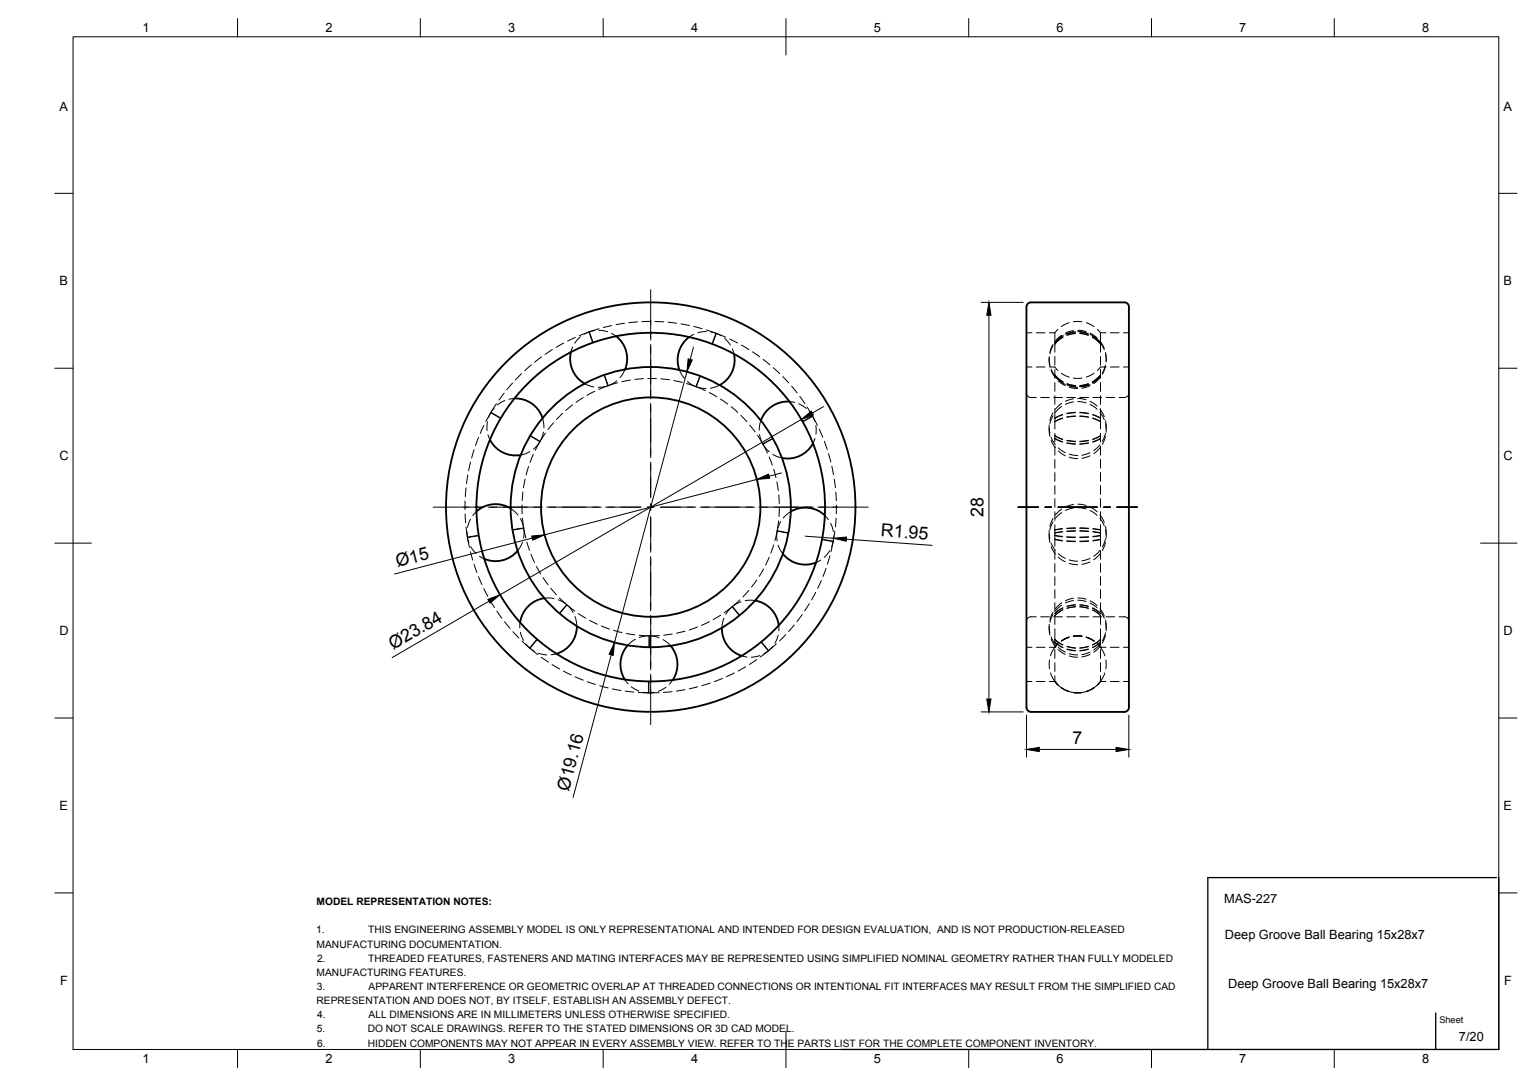
ISO-10303-21;
HEADER;
FILE_DESCRIPTION (('STEP AP214'),
    '1' );
FILE_NAME ( 'Deep Groove Ball Bearing 15x28x7.step', '2026-10-06T08:24:41', ( '' ), ( '' ), 'STEP AP214', 'Unspecified', '' );
FILE_SCHEMA (( 'AUTOMOTIVE_DESIGN' ));
ENDSEC;
DATA;
#5=EDGE_CURVE ( 'NONE', #3462, #12596, #11883, .T. ) ;
#6=CARTESIAN_POINT ( 'NONE',  ( 0.3607825703614780388, 0.06309631803704385256, 0.08455817587619855746 ) ) ;
#11=ORIENTED_EDGE ( 'NONE', *, *, #14941, .F. ) ;
#36=CARTESIAN_POINT ( 'NONE',  ( 0.4620608682196346573, 0.08206165078060492779, 0.1992125984251968684 ) ) ;
#61=AXIS2_PLACEMENT_3D ( 'NONE', #22056, #14008, #15706 ) ;
#62=CARTESIAN_POINT ( 'NONE',  ( 0.2428345617565153547, 0.2885915454824177218, 0.1992125984251968684 ) ) ;
#79=EDGE_LOOP ( 'NONE', ( #24549, #12991, #16155, #19629, #1630 ) ) ;
#92=DIRECTION ( 'NONE',  ( -0.8660254037844387076, 0.4999999999999998890, 0.000000000000000000 ) ) ;
#96=ORIENTED_EDGE ( 'NONE', *, *, #21914, .F. ) ;
#100=PRODUCT_DEFINITION_CONTEXT ( 'detailed design', #9805, 'design' ) ;
#103=CARTESIAN_POINT ( 'NONE',  ( 0.1669771619554775988, -0.4570419016558947556, 0.1827409795206137999 ) ) ;
#108=EDGE_LOOP ( 'NONE', ( #16831, #22102, #23011, #14973, #23434 ) ) ;
#112=AXIS2_PLACEMENT_3D ( 'NONE', #26701, #7362, #3107 ) ;
#125=DIRECTION ( 'NONE',  ( 0.000000000000000000, -1.000000000000000000, 0.000000000000000000 ) ) ;
#126=CARTESIAN_POINT ( 'NONE',  ( 0.0005789221761808661720, 0.4692909815006409691, 0.1992125984251968684 ) ) ;
#128=CARTESIAN_POINT ( 'NONE',  ( 0.000000000000000000, 0.000000000000000000, 0.01181102362204724393 ) ) ;
#135=ORIENTED_EDGE ( 'NONE', *, *, #15589, .F. ) ;
#137=DIRECTION ( 'NONE',  ( 0.000000000000000000, 0.000000000000000000, 1.000000000000000000 ) ) ;
#165=CARTESIAN_POINT ( 'NONE',  ( 0.000000000000000000, 0.000000000000000000, -3.278217716535432842E-17 ) ) ;
#169=EDGE_CURVE ( 'NONE', #21708, #16172, #21378, .T. ) ;
#182=CIRCLE ( 'NONE', #19069, 0.2952755905511810774 ) ;
#186=B_SPLINE_CURVE_WITH_KNOTS ( 'NONE', 3,
 ( #3405, #6229, #8475, #4376, #23337, #25576 ),
 .UNSPECIFIED., .F., .F.,
 ( 4, 2, 4 ),
 ( 0.2291966065698869959, 0.2305109203526899964, 0.2318252341354939960 ),
 .UNSPECIFIED. ) ;
#199=CARTESIAN_POINT ( 'NONE',  ( -0.3665264996331779601, -0.2116141732283464416, 0.1377952755905511861 ) ) ;
#211=EDGE_CURVE ( 'NONE', #8069, #8578, #17150, .T. ) ;
#222=SURFACE_STYLE_USAGE ( .BOTH. , #19537 ) ;
#226=CARTESIAN_POINT ( 'NONE',  ( 0.0005189969344232283309, 0.3771649972486724733, 0.07637795275590551769 ) ) ;
#230=ADVANCED_FACE ( 'NONE', ( #18229 ), #8731, .T. ) ;
#235=EDGE_CURVE ( 'NONE', #27620, #935, #8316, .T. ) ;
#237=FACE_OUTER_BOUND ( 'NONE', #646, .T. ) ;
#240=VERTEX_POINT ( 'NONE', #18659 ) ;
#243=FACE_OUTER_BOUND ( 'NONE', #27157, .T. ) ;
#251=EDGE_CURVE ( 'NONE', #10904, #1560, #4337, .T. ) ;
#256=DIRECTION ( 'NONE',  ( 0.000000000000000000, 0.000000000000000000, 1.000000000000000000 ) ) ;
#263=ORIENTED_EDGE ( 'NONE', *, *, #3631, .F. ) ;
#266=CIRCLE ( 'NONE', #11488, 0.4692913385826771866 ) ;
#286=B_SPLINE_CURVE_WITH_KNOTS ( 'NONE', 3,
 ( #23808, #10659, #8682, #25644, #1905, #25921 ),
 .UNSPECIFIED., .F., .F.,
 ( 4, 2, 4 ),
 ( 0.7157687286427140139, 0.7172350147555670574, 0.7187013008684199900 ),
 .UNSPECIFIED. ) ;
#308=DIRECTION ( 'NONE',  ( 0.7660444431189782355, 0.6427876096865391409, 0.000000000000000000 ) ) ;
#309=( CONVERSION_BASED_UNIT ( 'INCH', #689 ) LENGTH_UNIT ( ) NAMED_UNIT ( #9238 ) ) ;
#326=CARTESIAN_POINT ( 'NONE',  ( -0.1196556571310431333, -0.3272932875252256291, 0.1166443193928402983 ) ) ;
#339=VERTEX_POINT ( 'NONE', #12317 ) ;
#343=DIRECTION ( 'NONE',  ( 0.000000000000000000, 1.000000000000000000, 0.000000000000000000 ) ) ;
#355=EDGE_CURVE ( 'NONE', #14294, #8859, #26577, .T. ) ;
#365=CARTESIAN_POINT ( 'NONE',  ( 0.3411065095061437402, 0.06065137456822566192, 0.1377952755905510474 ) ) ;
#366=DIRECTION ( 'NONE',  ( 0.000000000000000000, 1.000000000000000000, 0.000000000000000000 ) ) ;
#367=AXIS2_PLACEMENT_3D ( 'NONE', #8300, #14535, #6190 ) ;
#370=ORIENTED_EDGE ( 'NONE', *, *, #13419, .F. ) ;
#385=CARTESIAN_POINT ( 'NONE',  ( -0.2230788859036006988, 0.2650812153444457309, 0.1276989850646860214 ) ) ;
#387=ORIENTED_EDGE ( 'NONE', *, *, #3265, .F. ) ;
#391=AXIS2_PLACEMENT_3D ( 'NONE', #18400, #12341, #14636 ) ;
#394=LINE ( 'NONE', #15375, #16281 ) ;
#404=VECTOR ( 'NONE', #11672, 39.37007874015748143 ) ;
#420=CARTESIAN_POINT ( 'NONE',  ( 0.3002886982018041495, -0.1727973894384573217, 0.1478915661278440430 ) ) ;
#421=TOROIDAL_SURFACE ( 'NONE', #8530, 0.4232283464566928832, 0.07677165354330708902 ) ;
#429=CIRCLE ( 'NONE', #27509, 0.07677362204724409722 ) ;
#435=DIRECTION ( 'NONE',  ( 0.000000000000000000, -1.000000000000000000, 0.000000000000000000 ) ) ;
#449=CARTESIAN_POINT ( 'NONE',  ( 0.3665264996331779601, -0.2116141732283464416, 0.06102165354330708891 ) ) ;
#451=CARTESIAN_POINT ( 'NONE',  ( 0.0003854097503897235258, 0.4692912202195575477, 0.07637630773773071424 ) ) ;
#457=AXIS2_PLACEMENT_3D ( 'NONE', #11632, #18253, #20541 ) ;
#484=CARTESIAN_POINT ( 'NONE',  ( 0.1706130639257694703, -0.4670119966460608563, 0.1140743250952255261 ) ) ;
#496=VERTEX_POINT ( 'NONE', #19091 ) ;
#497=CIRCLE ( 'NONE', #20352, 0.4692913385826771866 ) ;
#500=B_SPLINE_CURVE_WITH_KNOTS ( 'NONE', 3,
 ( #10699, #21447, #8173, #14554, #4212, #19314, #8315, #6201, #17200, #2088 ),
 .UNSPECIFIED., .F., .F.,
 ( 4, 2, 2, 2, 4 ),
 ( 0.000000000000000000, 0.2500000000000000000, 0.5000000000000000000, 0.7500000000000000000, 1.000000000000000000 ),
 .UNSPECIFIED. ) ;
#509=ADVANCED_FACE ( 'NONE', ( #25741, #6394 ), #27730, .T. ) ;
#515=DIRECTION ( 'NONE',  ( 0.000000000000000000, 1.000000000000000000, 0.000000000000000000 ) ) ;
#516=SHAPE_DEFINITION_REPRESENTATION ( #3947, #26684 ) ;
#551=CARTESIAN_POINT ( 'NONE',  ( 0.4061284506584276199, -0.2351468520616558922, 0.07637795275590551769 ) ) ;
#552=ORIENTED_EDGE ( 'NONE', *, *, #3585, .T. ) ;
#555=CARTESIAN_POINT ( 'NONE',  ( -0.4792984784078200833, 0.08391448672304414880, 0.09284957166327162392 ) ) ;
#559=CARTESIAN_POINT ( 'NONE',  ( -0.2420394123212937232, 0.2892587550802429575, 0.1992125984251968684 ) ) ;
#567=DIRECTION ( 'NONE',  ( 0.000000000000000000, 1.000000000000000000, 0.000000000000000000 ) ) ;
#573=FACE_BOUND ( 'NONE', #23313, .T. ) ;
#575=B_SPLINE_CURVE_WITH_KNOTS ( 'NONE', 3,
 ( #21559, #25522, #19016, #21142, #6187, #25800, #4193, #19296, #10823, #27882 ),
 .UNSPECIFIED., .F., .F.,
 ( 4, 2, 2, 2, 4 ),
 ( 0.000000000000000000, 0.2500000000000000000, 0.5000000000000000000, 0.7500000000000000000, 1.000000000000000000 ),
 .UNSPECIFIED. ) ;
#582=CARTESIAN_POINT ( 'NONE',  ( -0.1291602287245499914, -0.3543605079199910191, 0.07637549214372835182 ) ) ;
#584=DIRECTION ( 'NONE',  ( 0.000000000000000000, 0.000000000000000000, 1.000000000000000000 ) ) ;
#586=CIRCLE ( 'NONE', #13192, 0.3464566929133857665 ) ;
#596=B_SPLINE_CURVE_WITH_KNOTS ( 'NONE', 3,
 ( #25551, #6069, #1950, #3792, #12413, #10279 ),
 .UNSPECIFIED., .F., .F.,
 ( 4, 2, 4 ),
 ( 0.6902184472752670441, 0.6915327610580710438, 0.6928470748408740443 ),
 .UNSPECIFIED. ) ;
#602=CARTESIAN_POINT ( 'NONE',  ( 0.000000000000000000, 0.000000000000000000, 0.2637795275590551491 ) ) ;
#604=CARTESIAN_POINT ( 'NONE',  ( -0.4302903874076512425, -0.2491168502841591137, 0.1615162260931827798 ) ) ;
#608=EDGE_CURVE ( 'NONE', #21708, #2190, #18099, .T. ) ;
#610=CARTESIAN_POINT ( 'NONE',  ( 0.0005114926878545973925, 0.3662580330867914458, 0.1910323753037862504 ) ) ;
#613=CARTESIAN_POINT ( 'NONE',  ( 0.3714952424334504455, 0.06515381386493819538, 0.1992142436757342316 ) ) ;
#634=CARTESIAN_POINT ( 'NONE',  ( 0.3665264996331779601, -0.2116141732283464416, 0.2145688976377952695 ) ) ;
#635=ADVANCED_FACE ( 'NONE', ( #22183 ), #9450, .T. ) ;
#646=EDGE_LOOP ( 'NONE', ( #20143, #20285, #18872, #16802, #20608, #22874 ) ) ;
#658=ORIENTED_EDGE ( 'NONE', *, *, #21103, .T. ) ;
#661=VERTEX_POINT ( 'NONE', #24573 ) ;
#676=EDGE_CURVE ( 'NONE', #25669, #5138, #6693, .T. ) ;
#678=DIRECTION ( 'NONE',  ( 0.000000000000000000, 0.000000000000000000, 1.000000000000000000 ) ) ;
#687=AXIS2_PLACEMENT_3D ( 'NONE', #19653, #20189, #4936 ) ;
#689=LENGTH_MEASURE_WITH_UNIT ( LENGTH_MEASURE( 0.02539999999999999897 ), #14996 ) ;
#690=ORIENTED_EDGE ( 'NONE', *, *, #10619, .F. ) ;
#710=AXIS2_PLACEMENT_3D ( 'NONE', #24848, #16245, #9579 ) ;
#729=DIRECTION ( 'NONE',  ( 0.000000000000000000, 1.000000000000000000, 0.000000000000000000 ) ) ;
#735=CARTESIAN_POINT ( 'NONE',  ( 0.1447526197146039584, -0.3977045540727763839, 0.2145688976377952695 ) ) ;
#740=ORIENTED_EDGE ( 'NONE', *, *, #20229, .T. ) ;
#762=VERTEX_POINT ( 'NONE', #16114 ) ;
#764=VERTEX_POINT ( 'NONE', #8065 ) ;
#788=AXIS2_PLACEMENT_3D ( 'NONE', #5285, #22529, #17715 ) ;
#803=ORIENTED_EDGE ( 'NONE', *, *, #20955, .T. ) ;
#812=DIRECTION ( 'NONE',  ( 1.000000000000000000, 0.000000000000000000, 0.000000000000000000 ) ) ;
#820=DIRECTION ( 'NONE',  ( -0.9848077530122079093, 0.1736481776669309696, 0.000000000000000000 ) ) ;
#834=CARTESIAN_POINT ( 'NONE',  ( -0.4065144339881236468, -0.2344790234878192936, 0.07637549214372835182 ) ) ;
#835=ORIENTED_EDGE ( 'NONE', *, *, #3265, .T. ) ;
#845=CARTESIAN_POINT ( 'NONE',  ( 0.000000000000000000, 0.3771653543307086909, 0.2755905511811023723 ) ) ;
#848=DIRECTION ( 'NONE',  ( 0.000000000000000000, 0.000000000000000000, 1.000000000000000000 ) ) ;
#854=CARTESIAN_POINT ( 'NONE',  ( -0.1180276236025431108, -0.3257325899126714552, 0.1276989850612303967 ) ) ;
#881=ORIENTED_EDGE ( 'NONE', *, *, #14494, .F. ) ;
#884=CARTESIAN_POINT ( 'NONE',  ( -0.3105951325225213000, -0.1787383246545907467, 0.09506557084360875431 ) ) ;
#890=CARTESIAN_POINT ( 'NONE',  ( -0.3714653163189441387, 0.06532421472592696288, 0.07637549214372835182 ) ) ;
#916=DIRECTION ( 'NONE',  ( 0.000000000000000000, 0.000000000000000000, -1.000000000000000000 ) ) ;
#935=VERTEX_POINT ( 'NONE', #19202 ) ;
#946=EDGE_LOOP ( 'NONE', ( #5245, #370, #4472, #8238, #9152, #16696 ) ) ;
#954=DIRECTION ( 'NONE',  ( 0.000000000000000000, 1.000000000000000000, 0.000000000000000000 ) ) ;
#959=CARTESIAN_POINT ( 'NONE',  ( -0.4062254136079196942, -0.2349793847445165174, 0.1992142434433712694 ) ) ;
#986=CARTESIAN_POINT ( 'NONE',  ( 0.2230788859036007821, 0.2650812153444456198, 0.1377952755905513527 ) ) ;
#994=CARTESIAN_POINT ( 'NONE',  ( -0.1187185187216169419, -0.3276343780110584913, 0.1166443193947863527 ) ) ;
#997=DIRECTION ( 'NONE',  ( 0.000000000000000000, 0.000000000000000000, 1.000000000000000000 ) ) ;
#998=CARTESIAN_POINT ( 'NONE',  ( -0.3012109481301850633, 0.3598698725862389813, 0.07637795275590551769 ) ) ;
#1006=AXIS2_PLACEMENT_3D ( 'NONE', #24971, #1119, #11840 ) ;
#1036=CARTESIAN_POINT ( 'NONE',  ( 0.000000000000000000, 0.000000000000000000, 0.1992125984251968684 ) ) ;
#1049=CARTESIAN_POINT ( 'NONE',  ( -0.0003454908279975151160, 0.3771652360013086902, 0.07637630750536809898 ) ) ;
#1050=ORIENTED_EDGE ( 'NONE', *, *, #16246, .F. ) ;
#1055=FACE_BOUND ( 'NONE', #16566, .T. ) ;
#1085=VERTEX_POINT ( 'NONE', #2918 ) ;
#1119=DIRECTION ( 'NONE',  ( 0.3420201433256691570, 0.9396926207859084279, -0.000000000000000000 ) ) ;
#1122=EDGE_LOOP ( 'NONE', ( #10970, #9534, #26213, #4529, #19127, #25779 ) ) ;
#1134=EDGE_CURVE ( 'NONE', #2754, #5280, #13734, .T. ) ;
#1137=B_SPLINE_CURVE_WITH_KNOTS ( 'NONE', 3,
 ( #26836, #22317, #13559, #16110, #2949, #11581, #1140, #9447, #18338, #998 ),
 .UNSPECIFIED., .F., .F.,
 ( 4, 2, 2, 2, 4 ),
 ( 0.000000000000000000, 0.2500000000000000000, 0.5000000000000000000, 0.7500000000000000000, 1.000000000000000000 ),
 .UNSPECIFIED. ) ;
#1140=CARTESIAN_POINT ( 'NONE',  ( -0.3191377210036941414, 0.3812612458990542463, 0.1140743250907937795 ) ) ;
#1166=CARTESIAN_POINT ( 'NONE',  ( 0.000000000000000000, 0.000000000000000000, 0.1377952755905511584 ) ) ;
#1171=CARTESIAN_POINT ( 'NONE',  ( -0.1285103288269285327, -0.3545966721392122545, 0.1992125984251968684 ) ) ;
#1174=CARTESIAN_POINT ( 'NONE',  ( 0.1601448837025507554, -0.4411213145380000200, 0.07637630773773071424 ) ) ;
#1179=TOROIDAL_SURFACE ( 'NONE', #8830, 0.4232283464566928832, 0.07677165354330708902 ) ;
#1199=DIRECTION ( 'NONE',  ( -0.6427876096865393629, 0.7660444431189780135, 0.000000000000000000 ) ) ;
#1201=CARTESIAN_POINT ( 'NONE',  ( -0.2420394123212937232, 0.2892587550802429575, 0.1992125984251968684 ) ) ;
#1213=CARTESIAN_POINT ( 'NONE',  ( 0.000000000000000000, 0.000000000000000000, 0.2374015748031496065 ) ) ;
#1218=AXIS2_PLACEMENT_3D ( 'NONE', #22516, #18393, #22374 ) ;
#1219=EDGE_CURVE ( 'NONE', #15450, #13929, #14689, .T. ) ;
#1238=CARTESIAN_POINT ( 'NONE',  ( 0.2952755905511810774, 0.000000000000000000, 0.2637795275590551491 ) ) ;
#1247=LINE ( 'NONE', #7602, #6111 ) ;
#1255=CARTESIAN_POINT ( 'NONE',  ( 0.000000000000000000, 0.000000000000000000, 0.01181102362204724393 ) ) ;
#1273=CARTESIAN_POINT ( 'NONE',  ( 0.4167985568850881561, 0.07349283109919289847, 0.06102165354330708891 ) ) ;
#1284=ORIENTED_EDGE ( 'NONE', *, *, #15743, .T. ) ;
#1290=FACE_OUTER_BOUND ( 'NONE', #17007, .T. ) ;
#1306=CARTESIAN_POINT ( 'NONE',  ( 0.2421724791772047192, 0.2891474103999575052, 0.1992142436757342316 ) ) ;
#1318=ADVANCED_FACE ( 'NONE', ( #14391 ), #2030, .T. ) ;
#1324=CARTESIAN_POINT ( 'NONE',  ( -0.3002886982018051487, -0.1727973894384558229, 0.1377952755905512416 ) ) ;
#1327=ORIENTED_EDGE ( 'NONE', *, *, #24883, .T. ) ;
#1333=CARTESIAN_POINT ( 'NONE',  ( -0.2350342994822195442, 0.2808987121525407527, 0.1910323753003855540 ) ) ;
#1348=VERTEX_POINT ( 'NONE', #21008 ) ;
#1350=FACE_OUTER_BOUND ( 'NONE', #24867, .T. ) ;
#1352=ORIENTED_EDGE ( 'NONE', *, *, #11882, .T. ) ;
#1361=B_SPLINE_CURVE_WITH_KNOTS ( 'NONE', 3,
 ( #7535, #1049, #3140, #9640 ),
 .UNSPECIFIED., .F., .F.,
 ( 4, 4 ),
 ( 0.2291966065698869959, 0.2305109203526903294 ),
 .UNSPECIFIED. ) ;
#1371=EDGE_CURVE ( 'NONE', #12126, #25040, #6106, .T. ) ;
#1392=CARTESIAN_POINT ( 'NONE',  ( -0.3715251363271980245, 0.06498290224717540031, 0.1992125984251968684 ) ) ;
#1394=CARTESIAN_POINT ( 'NONE',  ( 0.4620608682196346573, 0.08206165078060492779, 0.1992125984251968684 ) ) ;
#1409=EDGE_CURVE ( 'NONE', #18722, #9569, #7421, .T. ) ;
#1414=DIRECTION ( 'NONE',  ( 1.000000000000000000, 0.000000000000000000, 0.000000000000000000 ) ) ;
#1415=EDGE_CURVE ( 'NONE', #3132, #19812, #19791, .T. ) ;
#1420=CARTESIAN_POINT ( 'NONE',  ( 0.000000000000000000, 0.000000000000000000, 0.1377952755905511861 ) ) ;
#1424=CARTESIAN_POINT ( 'NONE',  ( -0.0005963271530280589861, 0.4972008316414383566, 0.1615162260929405846 ) ) ;
#1431=EDGE_CURVE ( 'NONE', #19638, #3330, #1584, .T. ) ;
#1457=CARTESIAN_POINT ( 'NONE',  ( 0.2350342994834856425, 0.2808987121540589826, 0.08455817587923418477 ) ) ;
#1477=ORIENTED_EDGE ( 'NONE', *, *, #1134, .F. ) ;
#1480=CARTESIAN_POINT ( 'NONE',  ( 0.3715251363271980245, 0.06498290224717499786, 0.1992125984251968684 ) ) ;
#1500=DIRECTION ( 'NONE',  ( 0.000000000000000000, 0.000000000000000000, 1.000000000000000000 ) ) ;
#1511=ORIENTED_EDGE ( 'NONE', *, *, #15544, .T. ) ;
#1517=DIRECTION ( 'NONE',  ( 0.000000000000000000, 0.000000000000000000, -1.000000000000000000 ) ) ;
#1518=DIRECTION ( 'NONE',  ( 0.000000000000000000, 0.000000000000000000, 1.000000000000000000 ) ) ;
#1519=DIRECTION ( 'NONE',  ( 0.000000000000000000, 0.000000000000000000, 1.000000000000000000 ) ) ;
#1524=ORIENTED_EDGE ( 'NONE', *, *, #26785, .T. ) ;
#1535=EDGE_CURVE ( 'NONE', #4856, #13865, #15573, .T. ) ;
#1540=CARTESIAN_POINT ( 'NONE',  ( 0.0004974201395668343718, 0.3464563358313495489, 0.1276989850566408180 ) ) ;
#1554=EDGE_LOOP ( 'NONE', ( #11117, #19270 ) ) ;
#1559=DIRECTION ( 'NONE',  ( 1.224646799147353207E-16, 1.000000000000000000, -0.000000000000000000 ) ) ;
#1560=VERTEX_POINT ( 'NONE', #19724 ) ;
#1566=DIRECTION ( 'NONE',  ( 0.000000000000000000, 0.000000000000000000, -1.000000000000000000 ) ) ;
#1573=ORIENTED_EDGE ( 'NONE', *, *, #16459, .T. ) ;
#1584=CIRCLE ( 'NONE', #6558, 0.4692913385826771866 ) ;
#1588=AXIS2_PLACEMENT_3D ( 'NONE', #21238, #19108, #17001 ) ;
#1593=DIRECTION ( 'NONE',  ( 0.000000000000000000, 1.000000000000000000, 0.000000000000000000 ) ) ;
#1614=CIRCLE ( 'NONE', #25063, 0.3771653543307086909 ) ;
#1630=ORIENTED_EDGE ( 'NONE', *, *, #18890, .F. ) ;
#1637=VERTEX_POINT ( 'NONE', #16323 ) ;
#1640=DIRECTION ( 'NONE',  ( -0.1736481776669300814, 0.9848077530122080203, 0.000000000000000000 ) ) ;
#1648=CARTESIAN_POINT ( 'NONE',  ( 0.3191377210044040735, 0.3812612458998947962, 0.1140743250939253023 ) ) ;
#1660=EDGE_LOOP ( 'NONE', ( #6013, #15520, #22967, #15519, #15320, #14141, #22628, #12183, #8642, #1327, #3586, #8439, #26231 ) ) ;
#1661=AXIS2_PLACEMENT_3D ( 'NONE', #6156, #15392, #11060 ) ;
#1663=DIRECTION ( 'NONE',  ( 1.000000000000000000, 0.000000000000000000, 0.000000000000000000 ) ) ;
#1683=CARTESIAN_POINT ( 'NONE',  ( 0.000000000000000000, 0.4232283464566928832, 0.2755905511811023723 ) ) ;
#1705=DIRECTION ( 'NONE',  ( 0.000000000000000000, 0.000000000000000000, 1.000000000000000000 ) ) ;
#1737=ORIENTED_EDGE ( 'NONE', *, *, #24013, .T. ) ;
#1787=DIRECTION ( 'NONE',  ( 0.000000000000000000, 1.000000000000000000, 0.000000000000000000 ) ) ;
#1793=FACE_OUTER_BOUND ( 'NONE', #6745, .T. ) ;
#1798=CARTESIAN_POINT ( 'NONE',  ( -0.3019498226894488102, 0.3592501948414881796, 0.07637630773773090853 ) ) ;
#1799=DIRECTION ( 'NONE',  ( 0.000000000000000000, 0.000000000000000000, 1.000000000000000000 ) ) ;
#1801=EDGE_LOOP ( 'NONE', ( #9800, #18373 ) ) ;
#1811=ORIENTED_EDGE ( 'NONE', *, *, #169, .T. ) ;
#1819=CARTESIAN_POINT ( 'NONE',  ( 0.000000000000000000, 0.000000000000000000, 0.1992125984251968684 ) ) ;
#1825=PLANE ( 'NONE',  #7840 ) ;
#1847=DIRECTION ( 'NONE',  ( -1.000000000000000000, 1.224646799147353454E-16, 0.000000000000000000 ) ) ;
#1848=EDGE_LOOP ( 'NONE', ( #13711, #22030, #20883, #10591 ) ) ;
#1857=DIRECTION ( 'NONE',  ( 0.3420201433256691015, -0.9396926207859082059, 0.000000000000000000 ) ) ;
#1880=AXIS2_PLACEMENT_3D ( 'NONE', #20412, #18117, #5296 ) ;
#1888=LINE ( 'NONE', #27610, #24730 ) ;
#1905=CARTESIAN_POINT ( 'NONE',  ( -0.3013593406941685315, 0.3597456680659448791, 0.1992142434433716580 ) ) ;
#1910=EDGE_LOOP ( 'NONE', ( #18795, #3060, #19622, #12675 ) ) ;
#1913=CARTESIAN_POINT ( 'NONE',  ( 0.0003854097504292619937, 0.4692912202195575477, 0.1992142434433716580 ) ) ;
#1916=ORIENTED_EDGE ( 'NONE', *, *, #5024, .F. ) ;
#1936=CARTESIAN_POINT ( 'NONE',  ( 0.000000000000000000, 0.000000000000000000, 0.2637795275590551491 ) ) ;
#1947=ORIENTED_EDGE ( 'NONE', *, *, #9292, .F. ) ;
#1950=CARTESIAN_POINT ( 'NONE',  ( -0.3714054139060130044, 0.06566393819133267695, 0.1992150590373740204 ) ) ;
#1951=VERTEX_POINT ( 'NONE', #18020 ) ;
#1954=CARTESIAN_POINT ( 'NONE',  ( -0.1669771619560911358, -0.4570419016575711368, 0.1827409795183129182 ) ) ;
#1959=CARTESIAN_POINT ( 'NONE',  ( 0.0005114926878485707464, 0.3662580330841583853, 0.08455817587929100043 ) ) ;
#1961=CARTESIAN_POINT ( 'NONE',  ( 0.4895436826821757959, 0.08692528595281577564, 0.1615162260900951940 ) ) ;
#1973=EDGE_LOOP ( 'NONE', ( #20423, #21873, #19738, #3498, #20930 ) ) ;
#1975=CARTESIAN_POINT ( 'NONE',  ( 0.1285103288269283661, -0.3545966721392122545, 0.07637795275590551769 ) ) ;
#1983=EDGE_CURVE ( 'NONE', #26656, #2802, #10615, .T. ) ;
#1993=DIRECTION ( 'NONE',  ( -0.8660254037844388186, -0.4999999999999997780, 0.000000000000000000 ) ) ;
#1994=CARTESIAN_POINT ( 'NONE',  ( 0.4897507849252922818, 0.08575075074490855209, 0.1140743250802734171 ) ) ;
#2011=CARTESIAN_POINT ( 'NONE',  ( 0.1189624676717049440, -0.3253923344978161825, 0.1377952755905510474 ) ) ;
#2021=DIRECTION ( 'NONE',  ( 0.000000000000000000, 1.000000000000000000, 0.000000000000000000 ) ) ;
#2030=TOROIDAL_SURFACE ( 'NONE', #19168, 0.3070866141732283561, 0.01181102362204724393 ) ;
#2035=EDGE_CURVE ( 'NONE', #27384, #13133, #7268, .T. ) ;
#2041=CARTESIAN_POINT ( 'NONE',  ( -0.4922996667773635315, 0.08741303158497767956, 0.1496602734588148298 ) ) ;
#2042=CARTESIAN_POINT ( 'NONE',  ( -0.1606879121748897576, -0.4409237942971110380, 0.07637549214372835182 ) ) ;
#2061=CARTESIAN_POINT ( 'NONE',  ( 0.000000000000000000, 0.000000000000000000, -3.278217716535432842E-17 ) ) ;
#2071=ORIENTED_EDGE ( 'NONE', *, *, #12180, .F. ) ;
#2074=DIRECTION ( 'NONE',  ( 1.000000000000000000, 0.000000000000000000, 0.000000000000000000 ) ) ;
#2080=EDGE_LOOP ( 'NONE', ( #7272, #15062, #27209, #14683, #12115, #6957 ) ) ;
#2085=EDGE_CURVE ( 'NONE', #21339, #11020, #11517, .T. ) ;
#2088=CARTESIAN_POINT ( 'NONE',  ( -0.1599629598573265865, -0.4411872753632007926, 0.1992125984251968684 ) ) ;
#2092=ORIENTED_EDGE ( 'NONE', *, *, #12180, .T. ) ;
#2106=CIRCLE ( 'NONE', #21510, 0.4692913385826771866 ) ;
#2110=TOROIDAL_SURFACE ( 'NONE', #20597, 0.4232283464566928832, 0.07677165354330708902 ) ;
#2111=B_SPLINE_CURVE_WITH_KNOTS ( 'NONE', 3,
 ( #16128, #24724, #22619, #14740, #10455, #27279 ),
 .UNSPECIFIED., .F., .F.,
 ( 4, 2, 4 ),
 ( 0.5000000000000000000, 0.7500000000000000000, 1.000000000000000000 ),
 .UNSPECIFIED. ) ;
#2120=EDGE_LOOP ( 'NONE', ( #5122, #17750, #15437, #8046 ) ) ;
#2133=DIRECTION ( 'NONE',  ( 1.000000000000000000, 0.000000000000000000, 0.000000000000000000 ) ) ;
#2153=DIRECTION ( 'NONE',  ( 1.000000000000000000, 0.000000000000000000, 0.000000000000000000 ) ) ;
#2190=VERTEX_POINT ( 'NONE', #21015 ) ;
#2204=VERTEX_POINT ( 'NONE', #22715 ) ;
#2230=CARTESIAN_POINT ( 'NONE',  ( 0.3020979083622633565, 0.3591256245826334181, 0.07637795275590551769 ) ) ;
#2242=DIRECTION ( 'NONE',  ( 0.000000000000000000, 0.000000000000000000, 1.000000000000000000 ) ) ;
#2249=B_SPLINE_CURVE_WITH_KNOTS ( 'NONE', 3,
 ( #9499, #22373, #2857, #13896, #18094, #2996, #27040, #11628, #7394, #12055 ),
 .UNSPECIFIED., .F., .F.,
 ( 4, 2, 2, 2, 4 ),
 ( 0.000000000000000000, 0.2500000000000001665, 0.5000000000000003331, 0.7500000000000001110, 1.000000000000000000 ),
 .UNSPECIFIED. ) ;
#2271=FACE_BOUND ( 'NONE', #4134, .T. ) ;
#2277=CARTESIAN_POINT ( 'NONE',  ( -0.1610509776512037416, -0.4407912692718771175, 0.07637795275590551769 ) ) ;
#2286=CARTESIAN_POINT ( 'NONE',  ( 0.000000000000000000, 0.2952755905511810774, 0.01181102362204724393 ) ) ;
#2289=FILL_AREA_STYLE_COLOUR ( '', #8101 ) ;
#2310=AXIS2_PLACEMENT_3D ( 'NONE', #7416, #9240, #16044 ) ;
#2323=EDGE_CURVE ( 'NONE', #339, #1560, #6148, .T. ) ;
#2349=DIRECTION ( 'NONE',  ( 0.8660254037844390407, -0.4999999999999994449, 0.000000000000000000 ) ) ;
#2354=CARTESIAN_POINT ( 'NONE',  ( 0.3264619303874873313, -0.1888818218344748001, 0.1992142436757342316 ) ) ;
#2366=ORIENTED_EDGE ( 'NONE', *, *, #8607, .T. ) ;
#2374=EDGE_CURVE ( 'NONE', #14762, #24304, #24142, .T. ) ;
#2384=CARTESIAN_POINT ( 'NONE',  ( -0.4716107359537566324, 0.08256389912709830026, 0.08349695147708714738 ) ) ;
#2394=VERTEX_POINT ( 'NONE', #11079 ) ;
#2399=CARTESIAN_POINT ( 'NONE',  ( -0.2428345617565149384, 0.2885915454824177218, 0.1992125984251968684 ) ) ;
#2408=CARTESIAN_POINT ( 'NONE',  ( 0.0001924259990422818461, 0.4692913385826771866, 0.07637549214372835182 ) ) ;
#2426=CARTESIAN_POINT ( 'NONE',  ( -0.2952755905511810774, 3.688404729715453115E-17, 0.01181102362204724393 ) ) ;
#2430=DIRECTION ( 'NONE',  ( 1.000000000000000000, 0.000000000000000000, 0.000000000000000000 ) ) ;
#2435=CARTESIAN_POINT ( 'NONE',  ( 0.000000000000000000, 0.5511811023622047445, 0.01181102362204724393 ) ) ;
#2439=CARTESIAN_POINT ( 'NONE',  ( -0.4061284506583976994, -0.2351468520617070734, 0.1992125984251968684 ) ) ;
#2445=ADVANCED_FACE ( 'NONE', ( #243 ), #17833, .F. ) ;
#2450=CARTESIAN_POINT ( 'NONE',  ( -0.4714076450717002986, 0.08371568475170254597, 0.1920935997043449750 ) ) ;
#2461=B_SPLINE_CURVE_WITH_KNOTS ( 'NONE', 3,
 ( #17933, #7095, #884, #18216, #18063, #24872 ),
 .UNSPECIFIED., .F., .F.,
 ( 4, 2, 4 ),
 ( 0.000000000000000000, 0.2499999999999998890, 0.5000000000000000000 ),
 .UNSPECIFIED. ) ;
#2470=DIRECTION ( 'NONE',  ( 0.000000000000000000, 0.000000000000000000, 1.000000000000000000 ) ) ;
#2477=EDGE_CURVE ( 'NONE', #23407, #7809, #24171, .T. ) ;
#2482=CARTESIAN_POINT ( 'NONE',  ( 0.1189624676717049440, -0.3253923344978161825, 0.1377952755905510474 ) ) ;
#2488=ORIENTED_EDGE ( 'NONE', *, *, #3295, .T. ) ;
#2516=FACE_OUTER_BOUND ( 'NONE', #23288, .T. ) ;
#2522=VERTEX_POINT ( 'NONE', #2716 ) ;
#2532=EDGE_LOOP ( 'NONE', ( #7536, #5991 ) ) ;
#2539=ADVANCED_FACE ( 'NONE', ( #2271, #12732 ), #18948, .T. ) ;
#2542=FACE_OUTER_BOUND ( 'NONE', #3536, .T. ) ;
#2551=ORIENTED_EDGE ( 'NONE', *, *, #23911, .F. ) ;
#2563=CARTESIAN_POINT ( 'NONE',  ( -0.3268074212154853941, -0.1882834141668338901, 0.1992142436757342316 ) ) ;
#2565=( GEOMETRIC_REPRESENTATION_CONTEXT ( 3 ) GLOBAL_UNCERTAINTY_ASSIGNED_CONTEXT ( ( #14423 ) ) GLOBAL_UNIT_ASSIGNED_CONTEXT ( ( #309, #11554, #24143 ) ) REPRESENTATION_CONTEXT ( 'NONE', 'WORKASPACE' ) ) ;
#2574=EDGE_CURVE ( 'NONE', #18722, #496, #24781, .T. ) ;
#2575=CARTESIAN_POINT ( 'NONE',  ( 0.3082037322259243428, 0.3663931537943041494, 0.1920935997044755372 ) ) ;
#2583=DIRECTION ( 'NONE',  ( 0.4999999999999996114, 0.8660254037844389297, 0.000000000000000000 ) ) ;
#2591=VERTEX_POINT ( 'NONE', #19374 ) ;
#2601=CARTESIAN_POINT ( 'NONE',  ( -0.2243804351489621651, 0.2666304421170154759, 0.1166443193998331490 ) ) ;
#2611=ORIENTED_EDGE ( 'NONE', *, *, #15702, .F. ) ;
#2617=ADVANCED_FACE ( 'NONE', ( #25802, #23284 ), #27795, .T. ) ;
#2636=CARTESIAN_POINT ( 'NONE',  ( -0.4167985568850881561, 0.07349283109919310664, 0.1377952755905511861 ) ) ;
#2641=ORIENTED_EDGE ( 'NONE', *, *, #6158, .F. ) ;
#2647=AXIS2_PLACEMENT_3D ( 'NONE', #2061, #19434, #125 ) ;
#2648=CARTESIAN_POINT ( 'NONE',  ( -4.618943439303797186E-17, -0.3771653543307086909, 0.2755905511811023723 ) ) ;
#2658=CARTESIAN_POINT ( 'NONE',  ( -0.4897507849295944515, 0.08575075074566133881, 0.1140743250927050007 ) ) ;
#2666=ADVANCED_FACE ( 'NONE', ( #16628 ), #15675, .T. ) ;
#2668=AXIS2_PLACEMENT_3D ( 'NONE', #15432, #4402, #12870 ) ;
#2677=CARTESIAN_POINT ( 'NONE',  ( 0.0001724821237276073489, 0.3771653543307085243, 0.07637549214372833795 ) ) ;
#2680=CARTESIAN_POINT ( 'NONE',  ( -0.1285103288269285327, -0.3545966721392122545, 0.07637795275590551769 ) ) ;
#2693=AXIS2_PLACEMENT_3D ( 'NONE', #16720, #10352, #2021 ) ;
#2694=DIRECTION ( 'NONE',  ( 1.000000000000000000, 0.000000000000000000, 0.000000000000000000 ) ) ;
#2696=DIRECTION ( 'NONE',  ( 1.000000000000000000, 0.000000000000000000, 0.000000000000000000 ) ) ;
#2708=CARTESIAN_POINT ( 'NONE',  ( 0.3713752547280854133, 0.06583429795695137920, 0.1992142436757342316 ) ) ;
#2716=CARTESIAN_POINT ( 'NONE',  ( -0.3020979083623086536, 0.3591256245825952265, 0.1992125984251968684 ) ) ;
#2725=CARTESIAN_POINT ( 'NONE',  ( 0.2423050875943944527, 0.2890362931940642088, 0.07637549214372835182 ) ) ;
#2737=EDGE_LOOP ( 'NONE', ( #14308, #15198, #18817, #27078 ) ) ;
#2746=CYLINDRICAL_SURFACE ( 'NONE', #14802, 0.4692913385826771866 ) ;
#2753=B_SPLINE_CURVE_WITH_KNOTS ( 'NONE', 3,
 ( #8016, #16623, #21003, #1648, #10252, #8157, #16767, #11169, #21110, #18984 ),
 .UNSPECIFIED., .F., .F.,
 ( 4, 2, 2, 2, 4 ),
 ( 0.000000000000000000, 0.2500000000000000000, 0.5000000000000000000, 0.7500000000000000000, 1.000000000000000000 ),
 .UNSPECIFIED. ) ;
#2754=VERTEX_POINT ( 'NONE', #17045 ) ;
#2757=ORIENTED_EDGE ( 'NONE', *, *, #17561, .T. ) ;
#2780=CARTESIAN_POINT ( 'NONE',  ( 0.4211031283186273955, -0.2438048970108675773, 0.1827409795176048457 ) ) ;
#2793=ORIENTED_EDGE ( 'NONE', *, *, #23347, .F. ) ;
#2802=VERTEX_POINT ( 'NONE', #126 ) ;
#2804=CARTESIAN_POINT ( 'NONE',  ( 0.4065144339881236468, -0.2344790234878192936, 0.07637549214372854611 ) ) ;
#2810=DIRECTION ( 'NONE',  ( 0.000000000000000000, 0.000000000000000000, 1.000000000000000000 ) ) ;
#2819=CARTESIAN_POINT ( 'NONE',  ( 0.000000000000000000, 0.000000000000000000, 0.1377952755905511861 ) ) ;
#2825=CARTESIAN_POINT ( 'NONE',  ( -0.3263749705684267921, -0.1890319631540330891, 0.1992125984251968684 ) ) ;
#2828=AXIS2_PLACEMENT_3D ( 'NONE', #13039, #9067, #26302 ) ;
#2857=CARTESIAN_POINT ( 'NONE',  ( 0.4216927985368217335, -0.2427835582310488571, 0.09284957166208239465 ) ) ;
#2864=CARTESIAN_POINT ( 'NONE',  ( 0.000000000000000000, 0.000000000000000000, 0.2755905511811023723 ) ) ;
#2894=CARTESIAN_POINT ( 'NONE',  ( -0.1599629598573265865, -0.4411872753632007926, 0.1992125984251968684 ) ) ;
#2905=DIRECTION ( 'NONE',  ( 0.000000000000000000, 0.000000000000000000, -1.000000000000000000 ) ) ;
#2917=EDGE_CURVE ( 'NONE', #23029, #19454, #20648, .T. ) ;
#2918=CARTESIAN_POINT ( 'NONE',  ( 0.1599629598573263645, -0.4411872753632007926, 0.1992125984251968684 ) ) ;
#2921=CARTESIAN_POINT ( 'NONE',  ( 0.4302903874081785984, -0.2491168502844573474, 0.1140743250896437688 ) ) ;
#2936=DIRECTION ( 'NONE',  ( -0.9848077530122082424, -0.1736481776669300259, 0.000000000000000000 ) ) ;
#2949=CARTESIAN_POINT ( 'NONE',  ( -0.3209354104562381349, 0.3834063931592568419, 0.1496602734580050054 ) ) ;
#2974=DIRECTION ( 'NONE',  ( 1.000000000000000000, 0.000000000000000000, 0.000000000000000000 ) ) ;
#2978=AXIS2_PLACEMENT_3D ( 'NONE', #22942, #16569, #3559 ) ;
#2980=DIRECTION ( 'NONE',  ( 0.000000000000000000, 0.000000000000000000, 1.000000000000000000 ) ) ;
#2996=CARTESIAN_POINT ( 'NONE',  ( 0.4333114377122374572, -0.2494818589555374000, 0.1496602734576668314 ) ) ;
#2998=DIRECTION ( 'NONE',  ( 0.000000000000000000, 0.000000000000000000, 1.000000000000000000 ) ) ;
#3004=CARTESIAN_POINT ( 'NONE',  ( 0.000000000000000000, 0.000000000000000000, 0.07637795275590551769 ) ) ;
#3005=EDGE_CURVE ( 'NONE', #14102, #6801, #12966, .T. ) ;
#3030=CARTESIAN_POINT ( 'NONE',  ( 0.1291602287245497971, -0.3543605079199910191, 0.1992150590373740204 ) ) ;
#3038=FACE_OUTER_BOUND ( 'NONE', #25601, .T. ) ;
#3047=B_SPLINE_CURVE_WITH_KNOTS ( 'NONE', 3,
 ( #15958, #12272, #25128, #24558, #9578, #10015 ),
 .UNSPECIFIED., .F., .F.,
 ( 4, 2, 4 ),
 ( 0.7157687286427140139, 0.7172350147555670574, 0.7187013008684189908 ),
 .UNSPECIFIED. ) ;
#3054=TOROIDAL_SURFACE ( 'NONE', #18860, 0.4232283464566928832, 0.07677165354330708902 ) ;
#3060=ORIENTED_EDGE ( 'NONE', *, *, #11134, .T. ) ;
#3090=CARTESIAN_POINT ( 'NONE',  ( -0.1286734528930088550, -0.3545375539099149265, 0.07637630750536809898 ) ) ;
#3091=DIRECTION ( 'NONE',  ( 0.000000000000000000, 1.000000000000000000, 0.000000000000000000 ) ) ;
#3102=CARTESIAN_POINT ( 'NONE',  ( 0.000000000000000000, 0.000000000000000000, 0.2755905511811023723 ) ) ;
#3103=AXIS2_PLACEMENT_3D ( 'NONE', #25732, #1857, #21496 ) ;
#3107=DIRECTION ( 'NONE',  ( 0.000000000000000000, -1.000000000000000000, 0.000000000000000000 ) ) ;
#3116=B_SPLINE_CURVE_WITH_KNOTS ( 'NONE', 3,
 ( #10774, #17276, #11053, #10625, #19392, #13308 ),
 .UNSPECIFIED., .F., .F.,
 ( 4, 2, 4 ),
 ( 0.000000000000000000, 0.2500000000000000000, 0.5000000000000000000 ),
 .UNSPECIFIED. ) ;
#3132=VERTEX_POINT ( 'NONE', #22237 ) ;
#3136=CARTESIAN_POINT ( 'NONE',  ( 0.000000000000000000, 0.000000000000000000, 0.1377952755905511584 ) ) ;
#3139=AXIS2_PLACEMENT_3D ( 'NONE', #11704, #2936, #20846 ) ;
#3140=CARTESIAN_POINT ( 'NONE',  ( -0.0001724821237274320063, 0.3771653543307086909, 0.07637549214372835182 ) ) ;
#3144=CARTESIAN_POINT ( 'NONE',  ( -0.1608692170994283632, -0.4408576787418519993, 0.1992142434433716580 ) ) ;
#3179=EDGE_LOOP ( 'NONE', ( #24269, #12231, #18979, #26878, #16717, #1284, #25406, #4482, #12261, #20323, #15391, #27067, #5957 ) ) ;
#3181=FACE_BOUND ( 'NONE', #12605, .T. ) ;
#3213=VERTEX_POINT ( 'NONE', #26893 ) ;
#3217=CARTESIAN_POINT ( 'NONE',  ( 4.701028524955307180E-18, 0.4232283464566928832, 0.06102165354330708891 ) ) ;
#3227=CARTESIAN_POINT ( 'NONE',  ( -0.3263749705684267921, -0.1890319631540330891, 0.07637795275590551769 ) ) ;
#3233=AXIS2_PLACEMENT_3D ( 'NONE', #5793, #12422, #5933 ) ;
#3249=CARTESIAN_POINT ( 'NONE',  ( 0.000000000000000000, 0.3771653543307086909, 0.2374015748031496065 ) ) ;
#3253=DIRECTION ( 'NONE',  ( 0.000000000000000000, 0.000000000000000000, 1.000000000000000000 ) ) ;
#3265=EDGE_CURVE ( 'NONE', #5138, #26931, #25605, .T. ) ;
#3295=EDGE_CURVE ( 'NONE', #12667, #24639, #7116, .T. ) ;
#3305=CIRCLE ( 'NONE', #7399, 0.3070866141732283561 ) ;
#3327=AXIS2_PLACEMENT_3D ( 'NONE', #25026, #20652, #14305 ) ;
#3330=VERTEX_POINT ( 'NONE', #27325 ) ;
#3345=CARTESIAN_POINT ( 'NONE',  ( -0.0005789221761808661720, 0.4692909815006409691, 0.1992125984251968684 ) ) ;
#3352=ORIENTED_EDGE ( 'NONE', *, *, #1409, .F. ) ;
#3354=CARTESIAN_POINT ( 'NONE',  ( -0.2423050875943940918, 0.2890362931940642088, 0.1992150590373740204 ) ) ;
#3368=VERTEX_POINT ( 'NONE', #14337 ) ;
#3377=ORIENTED_EDGE ( 'NONE', *, *, #26972, .F. ) ;
#3380=( NAMED_UNIT ( * ) PLANE_ANGLE_UNIT ( ) SI_UNIT ( $, .RADIAN. ) ) ;
#3387=EDGE_CURVE ( 'NONE', #20876, #16172, #1888, .T. ) ;
#3390=VERTEX_POINT ( 'NONE', #10494 ) ;
#3395=DIRECTION ( 'NONE',  ( 1.000000000000000000, 0.000000000000000000, 0.000000000000000000 ) ) ;
#3405=CARTESIAN_POINT ( 'NONE',  ( 0.3268939675028499914, -0.1881330340946397728, 0.07637795275590551769 ) ) ;
#3407=ORIENTED_EDGE ( 'NONE', *, *, #1371, .F. ) ;
#3408=CIRCLE ( 'NONE', #7958, 0.4692913385826771866 ) ;
#3411=VERTEX_POINT ( 'NONE', #26035 ) ;
#3432=ORIENTED_EDGE ( 'NONE', *, *, #13391, .T. ) ;
#3445=B_SPLINE_CURVE_WITH_KNOTS ( 'NONE', 3,
 ( #24907, #14048, #16438, #26890, #7255, #9934 ),
 .UNSPECIFIED., .F., .F.,
 ( 4, 2, 4 ),
 ( 0.2291966065698869959, 0.2305109203526899964, 0.2318252341354939960 ),
 .UNSPECIFIED. ) ;
#3462=VERTEX_POINT ( 'NONE', #26169 ) ;
#3466=DIRECTION ( 'NONE',  ( 1.000000000000000000, 0.000000000000000000, 0.000000000000000000 ) ) ;
#3469=ADVANCED_FACE ( 'NONE', ( #17679 ), #10297, .F. ) ;
#3498=ORIENTED_EDGE ( 'NONE', *, *, #235, .T. ) ;
#3499=VERTEX_POINT ( 'NONE', #19809 ) ;
#3518=CARTESIAN_POINT ( 'NONE',  ( -3.616083068348483797E-17, -0.2952755905511810774, 0.01181102362204724393 ) ) ;
#3520=DIRECTION ( 'NONE',  ( 0.000000000000000000, 0.000000000000000000, 1.000000000000000000 ) ) ;
#3536=EDGE_LOOP ( 'NONE', ( #2757, #18553 ) ) ;
#3541=CARTESIAN_POINT ( 'NONE',  ( -0.1230388948648306058, -0.3365682031891569781, 0.1805249803386037022 ) ) ;
#3543=DIRECTION ( 'NONE',  ( 0.000000000000000000, 0.000000000000000000, -1.000000000000000000 ) ) ;
#3549=ORIENTED_EDGE ( 'NONE', *, *, #9458, .F. ) ;
#3559=DIRECTION ( 'NONE',  ( -0.4999999999999996114, 0.8660254037844389297, 0.000000000000000000 ) ) ;
#3560=CARTESIAN_POINT ( 'NONE',  ( 0.3015072509068775219, 0.3596217111730925509, 0.07637549214372835182 ) ) ;
#3567=CARTESIAN_POINT ( 'NONE',  ( 0.000000000000000000, 0.000000000000000000, 0.03818897637795275884 ) ) ;
#3580=ORIENTED_EDGE ( 'NONE', *, *, #17104, .T. ) ;
#3585=EDGE_CURVE ( 'NONE', #10706, #10366, #10435, .T. ) ;
#3586=ORIENTED_EDGE ( 'NONE', *, *, #19012, .T. ) ;
#3589=ORIENTED_EDGE ( 'NONE', *, *, #2917, .T. ) ;
#3609=CARTESIAN_POINT ( 'NONE',  ( 0.000000000000000000, 0.000000000000000000, 0.07637795275590551769 ) ) ;
#3631=EDGE_CURVE ( 'NONE', #240, #14102, #4294, .T. ) ;
#3643=CARTESIAN_POINT ( 'NONE',  ( 0.0005189969344232283309, 0.3771649972486724733, 0.07637795275590551769 ) ) ;
#3652=CARTESIAN_POINT ( 'NONE',  ( 0.000000000000000000, 0.4232283464566928832, 0.1377952755905511861 ) ) ;
#3662=EDGE_LOOP ( 'NONE', ( #25309, #5752, #22752, #9765, #6498, #1916, #18496, #8610 ) ) ;
#3663=AXIS2_PLACEMENT_3D ( 'NONE', #18497, #5815, #1847 ) ;
#3665=DIRECTION ( 'NONE',  ( 0.000000000000000000, 0.000000000000000000, 1.000000000000000000 ) ) ;
#3676=CIRCLE ( 'NONE', #20842, 0.07677362204724411110 ) ;
#3687=FACE_OUTER_BOUND ( 'NONE', #21920, .T. ) ;
#3692=CARTESIAN_POINT ( 'NONE',  ( 0.000000000000000000, 0.000000000000000000, 0.01181102362204724393 ) ) ;
#3705=CARTESIAN_POINT ( 'NONE',  ( 0.000000000000000000, 0.000000000000000000, 0.07637795275590551769 ) ) ;
#3709=VERTEX_POINT ( 'NONE', #17286 ) ;
#3731=ORIENTED_EDGE ( 'NONE', *, *, #16393, .T. ) ;
#3755=EDGE_CURVE ( 'NONE', #762, #6801, #12034, .T. ) ;
#3763=CIRCLE ( 'NONE', #13677, 0.5511811023622047445 ) ;
#3768=FACE_OUTER_BOUND ( 'NONE', #1973, .T. ) ;
#3770=FACE_BOUND ( 'NONE', #6327, .T. ) ;
#3771=FACE_OUTER_BOUND ( 'NONE', #19803, .T. ) ;
#3775=DIRECTION ( 'NONE',  ( 0.000000000000000000, 1.000000000000000000, 0.000000000000000000 ) ) ;
#3779=EDGE_LOOP ( 'NONE', ( #7984, #23776 ) ) ;
#3792=CARTESIAN_POINT ( 'NONE',  ( -0.3714653163189441387, 0.06532421472592696288, 0.1992150590373740204 ) ) ;
#3796=CIRCLE ( 'NONE', #15545, 0.4692913385826771866 ) ;
#3814=AXIS2_PLACEMENT_3D ( 'NONE', #9451, #7352, #3091 ) ;
#3842=DIRECTION ( 'NONE',  ( 0.000000000000000000, 0.000000000000000000, 1.000000000000000000 ) ) ;
#3847=EDGE_CURVE ( 'NONE', #8860, #3368, #16199, .T. ) ;
#3854=AXIS2_PLACEMENT_3D ( 'NONE', #1166, #22627, #5968 ) ;
#3872=CARTESIAN_POINT ( 'NONE',  ( -0.4061284506584276199, -0.2351468520616558922, 0.07637795275590551769 ) ) ;
#3877=CIRCLE ( 'NONE', #710, 0.4692913385826771866 ) ;
#3900=ADVANCED_FACE ( 'NONE', ( #22994 ), #20710, .F. ) ;
#3916=CARTESIAN_POINT ( 'NONE',  ( 0.000000000000000000, 0.000000000000000000, 0.1992125984251968684 ) ) ;
#3939=EDGE_LOOP ( 'NONE', ( #8054, #9658 ) ) ;
#3945=CARTESIAN_POINT ( 'NONE',  ( 0.4922996667774506840, 0.08741303158498647807, 0.1259302777228524794 ) ) ;
#3947=PRODUCT_DEFINITION_SHAPE ( 'NONE', 'NONE',  #16541 ) ;
#3979=DIRECTION ( 'NONE',  ( 0.000000000000000000, 0.000000000000000000, -1.000000000000000000 ) ) ;
#3982=CARTESIAN_POINT ( 'NONE',  ( -0.1189624676717059848, -0.3253923344978159604, 0.1377952755905513249 ) ) ;
#3985=B_SPLINE_CURVE_WITH_KNOTS ( 'NONE', 3,
 ( #20427, #7569, #17869, #17996 ),
 .UNSPECIFIED., .F., .F.,
 ( 4, 4 ),
 ( 0.6902184472752670441, 0.6915327610580708217 ),
 .UNSPECIFIED. ) ;
#3998=CIRCLE ( 'NONE', #21136, 0.2952755905511810774 ) ;
#4014=DIRECTION ( 'NONE',  ( 0.000000000000000000, 1.000000000000000000, 0.000000000000000000 ) ) ;
#4017=FACE_OUTER_BOUND ( 'NONE', #3179, .T. ) ;
#4044=CIRCLE ( 'NONE', #17972, 0.3771653543307086909 ) ;
#4047=CARTESIAN_POINT ( 'NONE',  ( 0.000000000000000000, 0.000000000000000000, 0.07637795275590551769 ) ) ;
#4071=ORIENTED_EDGE ( 'NONE', *, *, #7278, .F. ) ;
#4080=ORIENTED_EDGE ( 'NONE', *, *, #3585, .F. ) ;
#4116=CARTESIAN_POINT ( 'NONE',  ( 0.2307318466638932919, 0.2741888764671439604, 0.1805249803295128908 ) ) ;
#4120=ORIENTED_EDGE ( 'NONE', *, *, #15589, .T. ) ;
#4121=CARTESIAN_POINT ( 'NONE',  ( -0.1257482708739876276, -0.3439950301903625940, 0.08455817587927060008 ) ) ;
#4134=EDGE_LOOP ( 'NONE', ( #15243, #17542, #1947, #27532 ) ) ;
#4169=CARTESIAN_POINT ( 'NONE',  ( -0.4620608682196346573, 0.08206165078060512208, 0.1992125984251968684 ) ) ;
#4176=VECTOR ( 'NONE', #4885, 39.37007874015748143 ) ;
#4183=CARTESIAN_POINT ( 'NONE',  ( -0.4167985568850881561, 0.07349283109919310664, 0.1377952755905511861 ) ) ;
#4193=CARTESIAN_POINT ( 'NONE',  ( 0.0005963271530354272241, 0.4972008316437019904, 0.1140743250946049531 ) ) ;
#4204=EDGE_CURVE ( 'NONE', #23387, #7189, #11665, .T. ) ;
#4211=ORIENTED_EDGE ( 'NONE', *, *, #14748, .T. ) ;
#4212=CARTESIAN_POINT ( 'NONE',  ( -0.1704479274145711543, -0.4700505334971128990, 0.1259302777278768770 ) ) ;
#4229=ORIENTED_EDGE ( 'NONE', *, *, #19009, .F. ) ;
#4230=ADVANCED_FACE ( 'NONE', ( #1793 ), #22983, .T. ) ;
#4261=ORIENTED_EDGE ( 'NONE', *, *, #18963, .F. ) ;
#4263=CARTESIAN_POINT ( 'NONE',  ( -0.1230388948646404523, -0.3365682031886393366, 0.09506557084333611130 ) ) ;
#4264=DIRECTION ( 'NONE',  ( 0.000000000000000000, -1.000000000000000000, 0.000000000000000000 ) ) ;
#4266=CARTESIAN_POINT ( 'NONE',  ( 0.4167985568850881561, 0.07349283109919291235, 0.1377952755905511861 ) ) ;
#4267=DIRECTION ( 'NONE',  ( 0.000000000000000000, 0.000000000000000000, 1.000000000000000000 ) ) ;
#4279=CARTESIAN_POINT ( 'NONE',  ( 0.4620608682196457040, 0.08206165078054626638, 0.07637795275590551769 ) ) ;
#4294=LINE ( 'NONE', #26176, #14378 ) ;
#4296=AXIS2_PLACEMENT_3D ( 'NONE', #19164, #16774, #14955 ) ;
#4298=VERTEX_POINT ( 'NONE', #7880 ) ;
#4305=ADVANCED_FACE ( 'NONE', ( #3771 ), #9411, .F. ) ;
#4319=CARTESIAN_POINT ( 'NONE',  ( -0.3665264996331779601, -0.2116141732283464416, 0.1377952755905511861 ) ) ;
#4326=CARTESIAN_POINT ( 'NONE',  ( -0.2307318466648207722, 0.2741888764682436364, 0.09506557084940545077 ) ) ;
#4335=DIRECTION ( 'NONE',  ( 0.000000000000000000, 0.000000000000000000, 1.000000000000000000 ) ) ;
#4337=B_SPLINE_CURVE_WITH_KNOTS ( 'NONE', 3,
 ( #25030, #27296, #25315, #3541, #12170, #20655 ),
 .UNSPECIFIED., .F., .F.,
 ( 4, 2, 4 ),
 ( 0.5000000000000000000, 0.7500000000000000000, 1.000000000000000000 ),
 .UNSPECIFIED. ) ;
#4342=ADVANCED_FACE ( 'NONE', ( #14249, #25104 ), #13866, .T. ) ;
#4357=EDGE_LOOP ( 'NONE', ( #10983, #4487, #18521, #23672 ) ) ;
#4358=CARTESIAN_POINT ( 'NONE',  ( -0.1715719712210964643, -0.4696414150085483352, 0.1259302777219306335 ) ) ;
#4371=CYLINDRICAL_SURFACE ( 'NONE', #7410, 0.2952755905511810774 ) ;
#4374=ORIENTED_EDGE ( 'NONE', *, *, #5024, .T. ) ;
#4376=CARTESIAN_POINT ( 'NONE',  ( 0.3265485372158890010, -0.1887320510662011952, 0.07637549214372835182 ) ) ;
#4378=ORIENTED_EDGE ( 'NONE', *, *, #7794, .F. ) ;
#4386=EDGE_CURVE ( 'NONE', #2394, #3462, #4044, .T. ) ;
#4387=CARTESIAN_POINT ( 'NONE',  ( 0.3430989538744064205, 0.06100393589346814194, 0.1589462317967534899 ) ) ;
#4392=DIRECTION ( 'NONE',  ( 0.000000000000000000, 1.000000000000000000, 0.000000000000000000 ) ) ;
#4393=CARTESIAN_POINT ( 'NONE',  ( 0.1610509776512037416, -0.4407912692718771175, 0.07637795275590551769 ) ) ;
#4399=FACE_OUTER_BOUND ( 'NONE', #7120, .T. ) ;
#4402=DIRECTION ( 'NONE',  ( 0.000000000000000000, 0.000000000000000000, 1.000000000000000000 ) ) ;
#4404=CARTESIAN_POINT ( 'NONE',  ( -0.0003854097504293205949, 0.4692912202195575477, 0.1992142434433716580 ) ) ;
#4409=ORIENTED_EDGE ( 'NONE', *, *, #1431, .F. ) ;
#4419=ADVANCED_FACE ( 'NONE', ( #15291, #8902 ), #6247, .T. ) ;
#4422=CARTESIAN_POINT ( 'NONE',  ( 0.1230388948667837656, -0.3365682031944939867, 0.1805249803472324666 ) ) ;
#4423=EDGE_LOOP ( 'NONE', ( #3549, #11518, #17339, #23717, #25497, #2071, #23588, #11594, #16452, #3352, #5531, #4120, #96 ) ) ;
#4442=CARTESIAN_POINT ( 'NONE',  ( 0.1643029338975805220, -0.4497088275977013661, 0.08349695147766536540 ) ) ;
#4472=ORIENTED_EDGE ( 'NONE', *, *, #8181, .F. ) ;
#4482=ORIENTED_EDGE ( 'NONE', *, *, #5823, .T. ) ;
#4486=AXIS2_PLACEMENT_3D ( 'NONE', #12309, #16278, #5540 ) ;
#4487=ORIENTED_EDGE ( 'NONE', *, *, #3847, .F. ) ;
#4508=DIRECTION ( 'NONE',  ( 0.000000000000000000, 0.000000000000000000, 1.000000000000000000 ) ) ;
#4520=ORIENTED_EDGE ( 'NONE', *, *, #15404, .F. ) ;
#4529=ORIENTED_EDGE ( 'NONE', *, *, #13343, .F. ) ;
#4531=CARTESIAN_POINT ( 'NONE',  ( 0.2358179517464219221, 0.2802411498302517789, 0.08455817587866316931 ) ) ;
#4535=DIRECTION ( 'NONE',  ( 0.000000000000000000, 0.000000000000000000, 1.000000000000000000 ) ) ;
#4536=CARTESIAN_POINT ( 'NONE',  ( -0.0005056364805206488332, 0.3583524373864938606, 0.1805249803418977061 ) ) ;
#4539=CARTESIAN_POINT ( 'NONE',  ( -0.2423050875943940918, 0.2890362931940642088, 0.07637549214372854611 ) ) ;
#4555=ORIENTED_EDGE ( 'NONE', *, *, #16122, .T. ) ;
#4571=CARTESIAN_POINT ( 'NONE',  ( -0.4714076450717705757, 0.08371568475171299595, 0.08349695147681061858 ) ) ;
#4613=CARTESIAN_POINT ( 'NONE',  ( 0.3268074212154850611, -0.1882834141668342509, 0.1992142436757342316 ) ) ;
#4628=FACE_OUTER_BOUND ( 'NONE', #20418, .T. ) ;
#4633=EDGE_CURVE ( 'NONE', #16172, #8069, #14422, .T. ) ;
#4652=ORIENTED_EDGE ( 'NONE', *, *, #5150, .T. ) ;
#4654=CARTESIAN_POINT ( 'NONE',  ( 0.2230788859036007821, 0.2650812153444456198, 0.1377952755905513527 ) ) ;
#4656=CARTESIAN_POINT ( 'NONE',  ( 0.3012109481302311376, 0.3598698725862007897, 0.07637795275590551769 ) ) ;
#4657=AXIS2_PLACEMENT_3D ( 'NONE', #23628, #21498, #4264 ) ;
#4664=AXIS2_PLACEMENT_3D ( 'NONE', #17436, #24211, #26057 ) ;
#4667=DIRECTION ( 'NONE',  ( 0.000000000000000000, 0.000000000000000000, 1.000000000000000000 ) ) ;
#4678=ORIENTED_EDGE ( 'NONE', *, *, #6857, .T. ) ;
#4683=CARTESIAN_POINT ( 'NONE',  ( 0.000000000000000000, 0.000000000000000000, 0.1377952755905511861 ) ) ;
#4686=AXIS2_PLACEMENT_3D ( 'NONE', #10403, #2980, #24200 ) ;
#4691=DIRECTION ( 'NONE',  ( 0.000000000000000000, 0.000000000000000000, -1.000000000000000000 ) ) ;
#4702=CARTESIAN_POINT ( 'NONE',  ( 0.000000000000000000, 0.000000000000000000, 0.1377952755905511861 ) ) ;
#4707=DIRECTION ( 'NONE',  ( 0.8660254037844385966, -0.5000000000000000000, 0.000000000000000000 ) ) ;
#4716=ORIENTED_EDGE ( 'NONE', *, *, #16150, .F. ) ;
#4733=CARTESIAN_POINT ( 'NONE',  ( 0.000000000000000000, 0.000000000000000000, 0.1992125984251968684 ) ) ;
#4748=CIRCLE ( 'NONE', #1588, 0.3464566929133857665 ) ;
#4763=CARTESIAN_POINT ( 'NONE',  ( -0.5393700787401575214, 6.605378404849898113E-17, 0.01181102362204724393 ) ) ;
#4768=AXIS2_PLACEMENT_3D ( 'NONE', #13400, #21895, #435 ) ;
#4774=CARTESIAN_POINT ( 'NONE',  ( 0.4302903874092360303, -0.2491168502850711342, 0.1615162260879781098 ) ) ;
#4779=CARTESIAN_POINT ( 'NONE',  ( -0.4622619257814346572, 0.08092139668567638333, 0.07637795275590551769 ) ) ;
#4787=CARTESIAN_POINT ( 'NONE',  ( -0.1285103288269285327, -0.3545966721392122545, 0.07637795275590551769 ) ) ;
#4788=CIRCLE ( 'NONE', #19221, 0.3771653543307086909 ) ;
#4799=CARTESIAN_POINT ( 'NONE',  ( -0.3200513472070305454, 0.3804946224880222383, 0.1615162260920062487 ) ) ;
#4806=CARTESIAN_POINT ( 'NONE',  ( 0.000000000000000000, 0.000000000000000000, 0.07637795275590551769 ) ) ;
#4826=B_SPLINE_CURVE_WITH_KNOTS ( 'NONE', 3,
 ( #25756, #21789, #15034, #6681, #8785, #15173 ),
 .UNSPECIFIED., .F., .F.,
 ( 4, 2, 4 ),
 ( 0.000000000000000000, 0.2500000000000000000, 0.5000000000000000000 ),
 .UNSPECIFIED. ) ;
#4841=CIRCLE ( 'NONE', #7132, 0.3771653543307086909 ) ;
#4853=CARTESIAN_POINT ( 'NONE',  ( 0.2420394123212937232, 0.2892587550802425134, 0.07637795275590551769 ) ) ;
#4856=VERTEX_POINT ( 'NONE', #9984 ) ;
#4857=DIRECTION ( 'NONE',  ( 0.000000000000000000, -1.000000000000000000, 0.000000000000000000 ) ) ;
#4861=DIRECTION ( 'NONE',  ( 0.000000000000000000, 0.000000000000000000, 1.000000000000000000 ) ) ;
#4882=B_SPLINE_CURVE_WITH_KNOTS ( 'NONE', 3,
 ( #4169, #2450, #21958, #15190, #2041, #8945, #6427, #11205, #4571, #10654 ),
 .UNSPECIFIED., .F., .F.,
 ( 4, 2, 2, 2, 4 ),
 ( 0.000000000000000000, 0.2500000000000000000, 0.5000000000000000000, 0.7500000000000000000, 1.000000000000000000 ),
 .UNSPECIFIED. ) ;
#4885=DIRECTION ( 'NONE',  ( 0.000000000000000000, 0.000000000000000000, 1.000000000000000000 ) ) ;
#4889=ORIENTED_EDGE ( 'NONE', *, *, #27239, .F. ) ;
#4915=STYLED_ITEM ( 'NONE', ( #8655 ), #21329 ) ;
#4936=DIRECTION ( 'NONE',  ( 0.000000000000000000, 1.000000000000000000, 0.000000000000000000 ) ) ;
#4957=FACE_OUTER_BOUND ( 'NONE', #2080, .T. ) ;
#4964=CARTESIAN_POINT ( 'NONE',  ( -0.3264619303874877754, -0.1888818218344748001, 0.1992142436757342316 ) ) ;
#4967=DIRECTION ( 'NONE',  ( 0.000000000000000000, -1.000000000000000000, 0.000000000000000000 ) ) ;
#4977=DIRECTION ( 'NONE',  ( 0.000000000000000000, 0.000000000000000000, 1.000000000000000000 ) ) ;
#4992=ORIENTED_EDGE ( 'NONE', *, *, #18076, .F. ) ;
#5024=EDGE_CURVE ( 'NONE', #23096, #19036, #26141, .T. ) ;
#5032=DIRECTION ( 'NONE',  ( 0.1736481776669309696, 0.9848077530122079093, 0.000000000000000000 ) ) ;
#5033=EDGE_CURVE ( 'NONE', #20898, #22611, #3998, .T. ) ;
#5061=ORIENTED_EDGE ( 'NONE', *, *, #2374, .F. ) ;
#5066=DIRECTION ( 'NONE',  ( 1.000000000000000000, 0.000000000000000000, 0.000000000000000000 ) ) ;
#5069=TOROIDAL_SURFACE ( 'NONE', #20425, 0.4232283464566928832, 0.07677165354330708902 ) ;
#5073=FACE_OUTER_BOUND ( 'NONE', #17401, .T. ) ;
#5090=EDGE_CURVE ( 'NONE', #12575, #5387, #20154, .T. ) ;
#5102=TOROIDAL_SURFACE ( 'NONE', #9177, 0.4232283464566928832, 0.07677165354330708902 ) ;
#5110=ADVANCED_FACE ( 'NONE', ( #23069 ), #9372, .F. ) ;
#5118=EDGE_CURVE ( 'NONE', #11020, #16931, #18720, .T. ) ;
#5119=CARTESIAN_POINT ( 'NONE',  ( 0.1610509776512594748, -0.4407912692718567449, 0.1992125984251968684 ) ) ;
#5120=ORIENTED_EDGE ( 'NONE', *, *, #18963, .T. ) ;
#5122=ORIENTED_EDGE ( 'NONE', *, *, #5965, .F. ) ;
#5138=VERTEX_POINT ( 'NONE', #6122 ) ;
#5150=EDGE_CURVE ( 'NONE', #764, #2591, #20734, .T. ) ;
#5200=CARTESIAN_POINT ( 'NONE',  ( -0.3411065095061437957, 0.06065137456822555090, 0.1377952755905512139 ) ) ;
#5214=CARTESIAN_POINT ( 'NONE',  ( -0.1285103288269285327, -0.3545966721392122545, 0.07637795275590551769 ) ) ;
#5228=CARTESIAN_POINT ( 'NONE',  ( -0.2997912780622379314, -0.1736589463928940036, 0.1276989850587680886 ) ) ;
#5229=CARTESIAN_POINT ( 'NONE',  ( 0.000000000000000000, 0.000000000000000000, 0.000000000000000000 ) ) ;
#5238=ORIENTED_EDGE ( 'NONE', *, *, #16122, .F. ) ;
#5245=ORIENTED_EDGE ( 'NONE', *, *, #8116, .T. ) ;
#5259=EDGE_CURVE ( 'NONE', #19876, #1085, #8286, .T. ) ;
#5268=CARTESIAN_POINT ( 'NONE',  ( 0.3412792617076850221, 0.05967164814832588010, 0.1377952755905512139 ) ) ;
#5280=VERTEX_POINT ( 'NONE', #20765 ) ;
#5285=CARTESIAN_POINT ( 'NONE',  ( 0.000000000000000000, 0.000000000000000000, 0.2755905511811023723 ) ) ;
#5296=DIRECTION ( 'NONE',  ( 1.000000000000000000, 0.000000000000000000, 0.000000000000000000 ) ) ;
#5298=ORIENTED_EDGE ( 'NONE', *, *, #26389, .T. ) ;
#5316=DIRECTION ( 'NONE',  ( -0.9848077530122079093, 0.1736481776669309696, 0.000000000000000000 ) ) ;
#5345=VERTEX_POINT ( 'NONE', #10295 ) ;
#5365=ADVANCED_FACE ( 'NONE', ( #9008, #17761 ), #11685, .T. ) ;
#5387=VERTEX_POINT ( 'NONE', #24671 ) ;
#5416=B_SPLINE_CURVE_WITH_KNOTS ( 'NONE', 3,
 ( #9422, #22582, #24831, #12123, #9719, #18320 ),
 .UNSPECIFIED., .F., .F.,
 ( 4, 2, 4 ),
 ( 0.000000000000000000, 0.2500000000000000000, 0.5000000000000000000 ),
 .UNSPECIFIED. ) ;
#5428=CARTESIAN_POINT ( 'NONE',  ( -0.3268939675028499914, -0.1881330340946393564, 0.1992125984251968684 ) ) ;
#5437=DIRECTION ( 'NONE',  ( 0.000000000000000000, 0.000000000000000000, 1.000000000000000000 ) ) ;
#5478=EDGE_LOOP ( 'NONE', ( #6416, #14959, #835, #13822 ) ) ;
#5504=ORIENTED_EDGE ( 'NONE', *, *, #11101, .T. ) ;
#5505=DIRECTION ( 'NONE',  ( 0.000000000000000000, 0.000000000000000000, 1.000000000000000000 ) ) ;
#5514=CARTESIAN_POINT ( 'NONE',  ( 0.0003454908279976030448, 0.3771652360013086347, 0.07637630750536809898 ) ) ;
#5521=B_SPLINE_CURVE_WITH_KNOTS ( 'NONE', 3,
 ( #10894, #19509, #9040, #4539, #26275, #26010 ),
 .UNSPECIFIED., .F., .F.,
 ( 4, 2, 4 ),
 ( 0.2291966065698859967, 0.2305109203526899964, 0.2318252341354939960 ),
 .UNSPECIFIED. ) ;
#5525=AXIS2_PLACEMENT_3D ( 'NONE', #12862, #21491, #2133 ) ;
#5531=ORIENTED_EDGE ( 'NONE', *, *, #2574, .T. ) ;
#5540=DIRECTION ( 'NONE',  ( 0.000000000000000000, 1.000000000000000000, 0.000000000000000000 ) ) ;
#5542=DIRECTION ( 'NONE',  ( 0.000000000000000000, 1.000000000000000000, 0.000000000000000000 ) ) ;
#5544=VERTEX_POINT ( 'NONE', #26952 ) ;
#5595=ORIENTED_EDGE ( 'NONE', *, *, #8491, .F. ) ;
#5609=CARTESIAN_POINT ( 'NONE',  ( 0.3070866141732283561, 0.000000000000000000, 0.01181102362204724393 ) ) ;
#5625=EDGE_CURVE ( 'NONE', #10367, #23405, #19331, .T. ) ;
#5629=EDGE_LOOP ( 'NONE', ( #263, #5750, #23968, #18754, #6100, #16886, #18842, #7683, #18642, #4652, #14285, #12418, #11589, #13376 ) ) ;
#5644=CARTESIAN_POINT ( 'NONE',  ( 0.0004986409324224840142, 0.3484797321218875421, 0.1166443193928900224 ) ) ;
#5659=CARTESIAN_POINT ( 'NONE',  ( -0.2420394123212937232, 0.2892587550802429575, 0.07637795275590551769 ) ) ;
#5677=CARTESIAN_POINT ( 'NONE',  ( -0.0005963271530349164564, 0.4972008316437025455, 0.1140743250946061466 ) ) ;
#5692=CARTESIAN_POINT ( 'NONE',  ( -0.3105951325233360372, -0.1787383246550589000, 0.1805249803389203656 ) ) ;
#5708=CARTESIAN_POINT ( 'NONE',  ( -0.1247869790646078808, -0.3443449117933338188, 0.1910323753003610736 ) ) ;
#5709=CARTESIAN_POINT ( 'NONE',  ( -3.616083068348483797E-17, -0.2952755905511810774, 0.1377952755905511861 ) ) ;
#5711=ORIENTED_EDGE ( 'NONE', *, *, #9036, .F. ) ;
#5723=ADVANCED_FACE ( 'NONE', ( #3687 ), #27495, .F. ) ;
#5750=ORIENTED_EDGE ( 'NONE', *, *, #12274, .T. ) ;
#5752=ORIENTED_EDGE ( 'NONE', *, *, #10357, .F. ) ;
#5753=CARTESIAN_POINT ( 'NONE',  ( 0.0004974201395668471654, 0.3464563358313494934, 0.1377952755905513249 ) ) ;
#5768=CARTESIAN_POINT ( 'NONE',  ( 0.000000000000000000, 0.000000000000000000, 0.01181102362204724393 ) ) ;
#5772=CARTESIAN_POINT ( 'NONE',  ( 0.000000000000000000, 0.000000000000000000, 0.1992125984251968684 ) ) ;
#5775=ORIENTED_EDGE ( 'NONE', *, *, #13391, .F. ) ;
#5780=DIRECTION ( 'NONE',  ( 0.000000000000000000, 0.000000000000000000, 1.000000000000000000 ) ) ;
#5790=AXIS2_PLACEMENT_3D ( 'NONE', #17138, #21937, #11057 ) ;
#5791=DIRECTION ( 'NONE',  ( 0.000000000000000000, 0.000000000000000000, 1.000000000000000000 ) ) ;
#5793=CARTESIAN_POINT ( 'NONE',  ( 0.000000000000000000, 0.000000000000000000, 0.2755905511811023723 ) ) ;
#5802=AXIS2_PLACEMENT_3D ( 'NONE', #4047, #1500, #12653 ) ;
#5815=DIRECTION ( 'NONE',  ( 1.224646799147353207E-16, 1.000000000000000000, -0.000000000000000000 ) ) ;
#5823=EDGE_CURVE ( 'NONE', #13865, #3709, #24715, .T. ) ;
#5839=AXIS2_PLACEMENT_3D ( 'NONE', #6183, #12928, #15212 ) ;
#5845=( GEOMETRIC_REPRESENTATION_CONTEXT ( 3 ) GLOBAL_UNCERTAINTY_ASSIGNED_CONTEXT ( ( #9879 ) ) GLOBAL_UNIT_ASSIGNED_CONTEXT ( ( #9609, #3380, #14011 ) ) REPRESENTATION_CONTEXT ( 'NONE', 'WORKASPACE' ) ) ;
#5853=CARTESIAN_POINT ( 'NONE',  ( 0.3105951325274823871, -0.1787383246574437701, 0.09506557083491969096 ) ) ;
#5855=CARTESIAN_POINT ( 'NONE',  ( -0.0004974201395671521515, 0.3464563358313494934, 0.1377952755905512139 ) ) ;
#5867=ORIENTED_EDGE ( 'NONE', *, *, #7076, .T. ) ;
#5882=CARTESIAN_POINT ( 'NONE',  ( 0.3013593406941685315, 0.3597456680659448791, 0.1992142434433716580 ) ) ;
#5893=EDGE_CURVE ( 'NONE', #8859, #19876, #25740, .T. ) ;
#5924=AXIS2_PLACEMENT_3D ( 'NONE', #24217, #4857, #916 ) ;
#5928=CIRCLE ( 'NONE', #22609, 0.3771653543307086909 ) ;
#5933=DIRECTION ( 'NONE',  ( 0.000000000000000000, 1.000000000000000000, 0.000000000000000000 ) ) ;
#5936=ORIENTED_EDGE ( 'NONE', *, *, #1219, .F. ) ;
#5957=ORIENTED_EDGE ( 'NONE', *, *, #8181, .T. ) ;
#5964=CARTESIAN_POINT ( 'NONE',  ( 0.1180276236025431108, -0.3257325899126714552, 0.1377952755905513527 ) ) ;
#5965=EDGE_CURVE ( 'NONE', #14009, #3330, #16665, .T. ) ;
#5968=DIRECTION ( 'NONE',  ( 1.000000000000000000, 0.000000000000000000, 0.000000000000000000 ) ) ;
#5978=CIRCLE ( 'NONE', #23117, 0.4692913385826771866 ) ;
#5990=B_SPLINE_CURVE_WITH_KNOTS ( 'NONE', 3,
 ( #13119, #21746, #6127, #8879 ),
 .UNSPECIFIED., .F., .F.,
 ( 4, 4 ),
 ( 0.2390783382518553157, 0.2405446243645580073 ),
 .UNSPECIFIED. ) ;
#5991=ORIENTED_EDGE ( 'NONE', *, *, #18076, .T. ) ;
#6000=AXIS2_PLACEMENT_3D ( 'NONE', #3567, #6001, #14780 ) ;
#6001=DIRECTION ( 'NONE',  ( 0.000000000000000000, 0.000000000000000000, 1.000000000000000000 ) ) ;
#6013=ORIENTED_EDGE ( 'NONE', *, *, #16544, .T. ) ;
#6061=ORIENTED_EDGE ( 'NONE', *, *, #20955, .F. ) ;
#6064=AXIS2_PLACEMENT_3D ( 'NONE', #8374, #19665, #10761 ) ;
#6069=CARTESIAN_POINT ( 'NONE',  ( -0.3713752547280854133, 0.06583429795695157349, 0.1992142436757342316 ) ) ;
#6080=FACE_OUTER_BOUND ( 'NONE', #25450, .T. ) ;
#6096=DIRECTION ( 'NONE',  ( 0.000000000000000000, -1.000000000000000000, 0.000000000000000000 ) ) ;
#6098=CARTESIAN_POINT ( 'NONE',  ( 0.1286734528930086607, -0.3545375539099149265, 0.07637630750536809898 ) ) ;
#6100=ORIENTED_EDGE ( 'NONE', *, *, #27239, .T. ) ;
#6105=EDGE_LOOP ( 'NONE', ( #20563, #23978 ) ) ;
#6106=CIRCLE ( 'NONE', #4296, 0.2952755905511810774 ) ;
#6107=CARTESIAN_POINT ( 'NONE',  ( 0.000000000000000000, 0.4232283464566928832, 0.1377952755905511861 ) ) ;
#6108=CARTESIAN_POINT ( 'NONE',  ( 0.000000000000000000, 0.3771653543307086909, -3.278217716535432842E-17 ) ) ;
#6111=VECTOR ( 'NONE', #1519, 39.37007874015748143 ) ;
#6122=CARTESIAN_POINT ( 'NONE',  ( -0.2223167940359792594, 0.2657206863494902538, 0.1377952755905513249 ) ) ;
#6126=EDGE_CURVE ( 'NONE', #20180, #27117, #17109, .T. ) ;
#6127=CARTESIAN_POINT ( 'NONE',  ( -0.0003854097503898040820, 0.4692912202195576032, 0.07637630773773071424 ) ) ;
#6128=B_SPLINE_CURVE_WITH_KNOTS ( 'NONE', 3,
 ( #27320, #14776, #23382, #16573, #12337, #8392 ),
 .UNSPECIFIED., .F., .F.,
 ( 4, 2, 4 ),
 ( 0.5000000000000000000, 0.7500000000000000000, 1.000000000000000000 ),
 .UNSPECIFIED. ) ;
#6148=CIRCLE ( 'NONE', #10635, 0.3771653543307086909 ) ;
#6151=CYLINDRICAL_SURFACE ( 'NONE', #6000, 0.4692913385826771866 ) ;
#6154=B_SPLINE_CURVE_WITH_KNOTS ( 'NONE', 3,
 ( #16619, #25796, #19152, #25660, #27649, #8563 ),
 .UNSPECIFIED., .F., .F.,
 ( 4, 2, 4 ),
 ( 0.5000000000000000000, 0.7499999999999998890, 1.000000000000000000 ),
 .UNSPECIFIED. ) ;
#6155=EDGE_CURVE ( 'NONE', #23029, #25669, #5521, .T. ) ;
#6156=CARTESIAN_POINT ( 'NONE',  ( 0.000000000000000000, 0.000000000000000000, 0.01181102362204724393 ) ) ;
#6158=EDGE_CURVE ( 'NONE', #10366, #22192, #26418, .T. ) ;
#6160=AXIS2_PLACEMENT_3D ( 'NONE', #16630, #22854, #8164 ) ;
#6169=CARTESIAN_POINT ( 'NONE',  ( -0.1610509776512037416, -0.4407912692718771175, 0.07637795275590551769 ) ) ;
#6170=DIRECTION ( 'NONE',  ( 0.000000000000000000, -1.000000000000000000, 0.000000000000000000 ) ) ;
#6176=CARTESIAN_POINT ( 'NONE',  ( 0.4065144339881338054, -0.2344790234878023627, 0.1992150590373740204 ) ) ;
#6177=ORIENTED_EDGE ( 'NONE', *, *, #251, .T. ) ;
#6183=CARTESIAN_POINT ( 'NONE',  ( 0.000000000000000000, 0.000000000000000000, 0.2374015748031496065 ) ) ;
#6187=CARTESIAN_POINT ( 'NONE',  ( 0.0005980912172666611815, 0.4999996422861968659, 0.1496602734623769526 ) ) ;
#6190=DIRECTION ( 'NONE',  ( 1.000000000000000000, 0.000000000000000000, 0.000000000000000000 ) ) ;
#6192=FACE_OUTER_BOUND ( 'NONE', #22187, .T. ) ;
#6201=CARTESIAN_POINT ( 'NONE',  ( -0.1658689444480831165, -0.4574452598412719895, 0.1827409795211070442 ) ) ;
#6211=ORIENTED_EDGE ( 'NONE', *, *, #26649, .T. ) ;
#6212=ORIENTED_EDGE ( 'NONE', *, *, #12680, .F. ) ;
#6213=CARTESIAN_POINT ( 'NONE',  ( -0.1643029338972192277, -0.4497088275967213167, 0.1920935997042204635 ) ) ;
#6229=CARTESIAN_POINT ( 'NONE',  ( 0.3268074212154850611, -0.1882834141668338901, 0.07637630750536809898 ) ) ;
#6244=AXIS2_PLACEMENT_3D ( 'NONE', #14121, #9731, #19916 ) ;
#6247=SPHERICAL_SURFACE ( 'NONE', #3103, 0.07677362204724409722 ) ;
#6257=CARTESIAN_POINT ( 'NONE',  ( 0.000000000000000000, 0.000000000000000000, -3.278217716535432842E-17 ) ) ;
#6274=CARTESIAN_POINT ( 'NONE',  ( 0.2720459371704843088, 0.3242117229735830830, 0.1377952755905511861 ) ) ;
#6280=CARTESIAN_POINT ( 'NONE',  ( -0.4302903874097571135, -0.2491168502853802758, 0.1140743250948484666 ) ) ;
#6295=DIRECTION ( 'NONE',  ( 0.000000000000000000, 0.000000000000000000, 1.000000000000000000 ) ) ;
#6299=ORIENTED_EDGE ( 'NONE', *, *, #18379, .F. ) ;
#6309=DIRECTION ( 'NONE',  ( 1.000000000000000000, 0.000000000000000000, 0.000000000000000000 ) ) ;
#6315=DIRECTION ( 'NONE',  ( 0.000000000000000000, 0.000000000000000000, 1.000000000000000000 ) ) ;
#6327=EDGE_LOOP ( 'NONE', ( #22336, #8855, #27429, #8820 ) ) ;
#6334=B_SPLINE_CURVE_WITH_KNOTS ( 'NONE', 3,
 ( #11559, #9023, #19641, #20175, #19908, #7055 ),
 .UNSPECIFIED., .F., .F.,
 ( 4, 2, 4 ),
 ( 0.000000000000000000, 0.2500000000000000000, 0.5000000000000000000 ),
 .UNSPECIFIED. ) ;
#6343=ORIENTED_EDGE ( 'NONE', *, *, #23489, .T. ) ;
#6350=CARTESIAN_POINT ( 'NONE',  ( 0.4790936880891605854, 0.08507591033000294622, 0.1827409795187460162 ) ) ;
#6361=EDGE_CURVE ( 'NONE', #17458, #16146, #16682, .T. ) ;
#6379=CARTESIAN_POINT ( 'NONE',  ( 0.000000000000000000, 0.000000000000000000, 0.1992125984251968684 ) ) ;
#6380=CARTESIAN_POINT ( 'NONE',  ( -0.0004986409324254199252, 0.3484797321232486755, 0.1589462317930222524 ) ) ;
#6381=DIRECTION ( 'NONE',  ( 0.000000000000000000, 0.000000000000000000, 1.000000000000000000 ) ) ;
#6384=DIRECTION ( 'NONE',  ( 1.000000000000000000, 0.000000000000000000, 0.000000000000000000 ) ) ;
#6394=FACE_OUTER_BOUND ( 'NONE', #18086, .T. ) ;
#6395=ORIENTED_EDGE ( 'NONE', *, *, #22413, .T. ) ;
#6403=FACE_OUTER_BOUND ( 'NONE', #12783, .T. ) ;
#6416=ORIENTED_EDGE ( 'NONE', *, *, #25747, .T. ) ;
#6427=CARTESIAN_POINT ( 'NONE',  ( -0.4895436826823449938, 0.08692528595285195503, 0.1140743250914997425 ) ) ;
#6440=DIRECTION ( 'NONE',  ( 0.000000000000000000, 1.000000000000000000, 0.000000000000000000 ) ) ;
#6462=ORIENTED_EDGE ( 'NONE', *, *, #11193, .F. ) ;
#6498=ORIENTED_EDGE ( 'NONE', *, *, #11729, .F. ) ;
#6558=AXIS2_PLACEMENT_3D ( 'NONE', #3916, #8435, #21152 ) ;
#6563=VERTEX_POINT ( 'NONE', #20121 ) ;
#6564=CIRCLE ( 'NONE', #3854, 0.3464566929133857665 ) ;
#6594=VERTEX_POINT ( 'NONE', #9706 ) ;
#6597=CARTESIAN_POINT ( 'NONE',  ( 0.3432721300525757857, 0.06002180498097315492, 0.1166443193853626548 ) ) ;
#6604=EDGE_LOOP ( 'NONE', ( #15331, #13608 ) ) ;
#6609=DIRECTION ( 'NONE',  ( -0.7660444431189780135, -0.6427876096865392519, 0.000000000000000000 ) ) ;
#6630=VERTEX_POINT ( 'NONE', #3518 ) ;
#6636=CIRCLE ( 'NONE', #1661, 0.5511811023622047445 ) ;
#6663=CARTESIAN_POINT ( 'NONE',  ( -0.2420394123212937232, 0.2892587550802429575, 0.07637795275590551769 ) ) ;
#6666=CARTESIAN_POINT ( 'NONE',  ( -1.456051859514965975E-17, 0.4692913385826771866, 0.1992150590373740204 ) ) ;
#6668=CARTESIAN_POINT ( 'NONE',  ( -0.3200513472080661614, 0.3804946224892518103, 0.1140743250936718939 ) ) ;
#6681=CARTESIAN_POINT ( 'NONE',  ( -0.2243804351500972571, 0.2666304421183634532, 0.1589462317874973663 ) ) ;
#6683=AXIS2_PLACEMENT_3D ( 'NONE', #8488, #27854, #17112 ) ;
#6686=DIRECTION ( 'NONE',  ( -0.4999999999999996114, -0.8660254037844389297, 0.000000000000000000 ) ) ;
#6688=FACE_OUTER_BOUND ( 'NONE', #17979, .T. ) ;
#6691=CARTESIAN_POINT ( 'NONE',  ( -0.4327133464943124785, -0.2505177833310021085, 0.1496602734626562570 ) ) ;
#6693=B_SPLINE_CURVE_WITH_KNOTS ( 'NONE', 3,
 ( #5659, #18341, #20628, #14136, #24708, #14283 ),
 .UNSPECIFIED., .F., .F.,
 ( 4, 2, 4 ),
 ( 0.000000000000000000, 0.2500000000000000000, 0.5000000000000000000 ),
 .UNSPECIFIED. ) ;
#6699=EDGE_CURVE ( 'NONE', #2591, #19036, #24790, .T. ) ;
#6700=CARTESIAN_POINT ( 'NONE',  ( 0.1610509776512037416, -0.4407912692718771175, 0.07637795275590551769 ) ) ;
#6728=CARTESIAN_POINT ( 'NONE',  ( -0.2358179517434294548, 0.2802411498267050605, 0.08455817588214351033 ) ) ;
#6745=EDGE_LOOP ( 'NONE', ( #2551, #11655, #26223, #1573, #16919 ) ) ;
#6760=ORIENTED_EDGE ( 'NONE', *, *, #27826, .F. ) ;
#6774=ADVANCED_FACE ( 'NONE', ( #20471 ), #16257, .F. ) ;
#6779=AXIS2_PLACEMENT_3D ( 'NONE', #9160, #22304, #11563 ) ;
#6780=EDGE_LOOP ( 'NONE', ( #5061, #4071, #26309, #11047 ) ) ;
#6794=DIRECTION ( 'NONE',  ( 0.000000000000000000, 1.000000000000000000, 0.000000000000000000 ) ) ;
#6795=FACE_BOUND ( 'NONE', #27723, .T. ) ;
#6798=DIRECTION ( 'NONE',  ( -0.8660254037844390407, -0.4999999999999994449, 0.000000000000000000 ) ) ;
#6801=VERTEX_POINT ( 'NONE', #845 ) ;
#6816=CARTESIAN_POINT ( 'NONE',  ( 0.1294857240059045234, -0.3542416573274181357, 0.1992125984251968684 ) ) ;
#6818=CARTESIAN_POINT ( 'NONE',  ( 0.3528204557988524614, 0.06272520244146252699, 0.09506557083424545251 ) ) ;
#6823=LENGTH_MEASURE_WITH_UNIT ( LENGTH_MEASURE( 0.02539999999999999897 ), #23922 ) ;
#6840=EDGE_LOOP ( 'NONE', ( #19040, #9763, #16834, #9950 ) ) ;
#6853=DIRECTION ( 'NONE',  ( 0.9396926207859082059, 0.3420201433256690460, 0.000000000000000000 ) ) ;
#6857=EDGE_CURVE ( 'NONE', #9819, #23096, #26713, .T. ) ;
#6867=ORIENTED_EDGE ( 'NONE', *, *, #18492, .T. ) ;
#6875=AXIS2_PLACEMENT_3D ( 'NONE', #23443, #10701, #15103 ) ;
#6901=CIRCLE ( 'NONE', #19971, 0.3771653543307086909 ) ;
#6916=DIRECTION ( 'NONE',  ( 0.6427876096865391409, -0.7660444431189782355, 0.000000000000000000 ) ) ;
#6924=EDGE_LOOP ( 'NONE', ( #9104, #18424 ) ) ;
#6930=EDGE_LOOP ( 'NONE', ( #8953, #14362 ) ) ;
#6956=CARTESIAN_POINT ( 'NONE',  ( 0.000000000000000000, 0.4232283464566928832, 0.1377952755905511861 ) ) ;
#6957=ORIENTED_EDGE ( 'NONE', *, *, #5033, .F. ) ;
#6964=EDGE_CURVE ( 'NONE', #10366, #20882, #18007, .T. ) ;
#6968=AXIS2_PLACEMENT_3D ( 'NONE', #4319, #18763, #20758 ) ;
#6983=CARTESIAN_POINT ( 'NONE',  ( -0.4067073728345788064, -0.2341441294389334793, 0.1992125984251968684 ) ) ;
#7005=AXIS2_PLACEMENT_3D ( 'NONE', #24131, #23997, #26117 ) ;
#7016=B_SPLINE_CURVE_WITH_KNOTS ( 'NONE', 3,
 ( #13026, #10910, #13305, #19532, #21930, #4279 ),
 .UNSPECIFIED., .F., .F.,
 ( 4, 2, 4 ),
 ( 0.2376120521391529850, 0.2390783382518550104, 0.2405446243645580073 ),
 .UNSPECIFIED. ) ;
#7032=CARTESIAN_POINT ( 'NONE',  ( 0.000000000000000000, 0.000000000000000000, 0.1992125984251968684 ) ) ;
#7055=CARTESIAN_POINT ( 'NONE',  ( -0.3411065095061437957, 0.06065137456822555090, 0.1377952755905512139 ) ) ;
#7076=EDGE_CURVE ( 'NONE', #21302, #21339, #20095, .T. ) ;
#7080=CARTESIAN_POINT ( 'NONE',  ( 0.000000000000000000, 0.000000000000000000, 0.2637795275590551491 ) ) ;
#7095=CARTESIAN_POINT ( 'NONE',  ( -0.3174445073348015067, -0.1826860508804799832, 0.08455817587939960800 ) ) ;
#7116=CIRCLE ( 'NONE', #391, 0.3464566929133857665 ) ;
#7120=EDGE_LOOP ( 'NONE', ( #740, #15771, #18224, #16093 ) ) ;
#7132=AXIS2_PLACEMENT_3D ( 'NONE', #13136, #17519, #6794 ) ;
#7134=FACE_OUTER_BOUND ( 'NONE', #27240, .T. ) ;
#7154=EDGE_LOOP ( 'NONE', ( #5120, #7356, #26951, #7279, #1477 ) ) ;
#7176=B_SPLINE_CURVE_WITH_KNOTS ( 'NONE', 3,
 ( #9882, #24853, #15692, #2804, #26542, #12007 ),
 .UNSPECIFIED., .F., .F.,
 ( 4, 2, 4 ),
 ( 0.2376120521391529850, 0.2390783382518560096, 0.2405446243645580073 ),
 .UNSPECIFIED. ) ;
#7178=EDGE_LOOP ( 'NONE', ( #23080, #658, #20468, #4678 ) ) ;
#7180=CARTESIAN_POINT ( 'NONE',  ( 0.4143458349590511403, -0.2398979215377306518, 0.1920935997039191212 ) ) ;
#7189=VERTEX_POINT ( 'NONE', #2230 ) ;
#7212=CIRCLE ( 'NONE', #112, 0.3070866141732283561 ) ;
#7236=CARTESIAN_POINT ( 'NONE',  ( 0.3200513472077004540, 0.3804946224888235418, 0.1140743250920687596 ) ) ;
#7255=CARTESIAN_POINT ( 'NONE',  ( 0.3714952424334504455, 0.06515381386493819538, 0.07637630750536809898 ) ) ;
#7257=FACE_OUTER_BOUND ( 'NONE', #27624, .T. ) ;
#7268=B_SPLINE_CURVE_WITH_KNOTS ( 'NONE', 3,
 ( #22288, #7180, #2780, #4774, #24268, #22021, #2921, #19760, #9014, #551 ),
 .UNSPECIFIED., .F., .F.,
 ( 4, 2, 2, 2, 4 ),
 ( 0.000000000000000000, 0.2500000000000000000, 0.5000000000000000000, 0.7500000000000000000, 1.000000000000000000 ),
 .UNSPECIFIED. ) ;
#7272=ORIENTED_EDGE ( 'NONE', *, *, #11101, .F. ) ;
#7275=CARTESIAN_POINT ( 'NONE',  ( 0.4620608682196346573, 0.08206165078060492779, 0.1992125984251968684 ) ) ;
#7278=EDGE_CURVE ( 'NONE', #20882, #14762, #16087, .T. ) ;
#7279=ORIENTED_EDGE ( 'NONE', *, *, #19009, .T. ) ;
#7338=DIRECTION ( 'NONE',  ( 0.000000000000000000, 0.000000000000000000, 1.000000000000000000 ) ) ;
#7348=DIRECTION ( 'NONE',  ( 1.000000000000000000, 0.000000000000000000, 0.000000000000000000 ) ) ;
#7350=DIRECTION ( 'NONE',  ( 0.000000000000000000, 0.000000000000000000, 1.000000000000000000 ) ) ;
#7352=DIRECTION ( 'NONE',  ( 0.000000000000000000, 0.000000000000000000, 1.000000000000000000 ) ) ;
#7355=ORIENTED_EDGE ( 'NONE', *, *, #25408, .T. ) ;
#7356=ORIENTED_EDGE ( 'NONE', *, *, #23911, .T. ) ;
#7362=DIRECTION ( 'NONE',  ( 0.000000000000000000, 0.000000000000000000, 1.000000000000000000 ) ) ;
#7369=DIRECTION ( 'NONE',  ( 0.000000000000000000, 0.000000000000000000, 1.000000000000000000 ) ) ;
#7375=AXIS2_PLACEMENT_3D ( 'NONE', #20025, #678, #9266 ) ;
#7376=DIRECTION ( 'NONE',  ( 0.000000000000000000, 0.000000000000000000, -1.000000000000000000 ) ) ;
#7392=AXIS2_PLACEMENT_3D ( 'NONE', #7080, #11041, #13151 ) ;
#7394=CARTESIAN_POINT ( 'NONE',  ( 0.4149306118460625581, -0.2388850582578112280, 0.1920935997041153531 ) ) ;
#7396=DIRECTION ( 'NONE',  ( 0.000000000000000000, -1.000000000000000000, 0.000000000000000000 ) ) ;
#7399=AXIS2_PLACEMENT_3D ( 'NONE', #14661, #2998, #7396 ) ;
#7410=AXIS2_PLACEMENT_3D ( 'NONE', #26509, #2242, #15127 ) ;
#7416=CARTESIAN_POINT ( 'NONE',  ( 0.000000000000000000, 0.000000000000000000, 0.2755905511811023723 ) ) ;
#7421=CIRCLE ( 'NONE', #18712, 0.4692913385826771866 ) ;
#7428=ADVANCED_FACE ( 'NONE', ( #15782, #3181 ), #9397, .T. ) ;
#7472=CARTESIAN_POINT ( 'NONE',  ( 0.2230788859036007821, 0.2650812153444456754, 0.1276989850664093651 ) ) ;
#7478=B_SPLINE_CURVE_WITH_KNOTS ( 'NONE', 3,
 ( #21464, #16801, #14567, #12968, #3945, #14712, #1961, #6350, #23593, #36 ),
 .UNSPECIFIED., .F., .F.,
 ( 4, 2, 2, 2, 4 ),
 ( 0.000000000000000000, 0.2500000000000001665, 0.5000000000000003331, 0.7500000000000001110, 1.000000000000000000 ),
 .UNSPECIFIED. ) ;
#7491=EDGE_CURVE ( 'NONE', #24053, #26265, #10399, .T. ) ;
#7496=CARTESIAN_POINT ( 'NONE',  ( 0.1447526197146039584, -0.3977045540727763839, 0.1377952755905511861 ) ) ;
#7525=CIRCLE ( 'NONE', #9842, 0.3771653543307086909 ) ;
#7534=VERTEX_POINT ( 'NONE', #21134 ) ;
#7535=CARTESIAN_POINT ( 'NONE',  ( -0.0005189969344232283309, 0.3771649972486724733, 0.07637795275590551769 ) ) ;
#7536=ORIENTED_EDGE ( 'NONE', *, *, #11302, .F. ) ;
#7537=CARTESIAN_POINT ( 'NONE',  ( -0.4149306118455106107, -0.2388850582574924275, 0.1920935997045936094 ) ) ;
#7538=CARTESIAN_POINT ( 'NONE',  ( -0.1601448837025137850, -0.4411213145380133982, 0.1992142434433712694 ) ) ;
#7568=CARTESIAN_POINT ( 'NONE',  ( 0.1288360683667812978, -0.3544784926413480086, 0.1992150590373740204 ) ) ;
#7569=CARTESIAN_POINT ( 'NONE',  ( 0.0003454908279975884623, 0.3771652360013086902, 0.1992142436757342316 ) ) ;
#7594=SPHERICAL_SURFACE ( 'NONE', #14266, 0.07677362204724409722 ) ;
#7602=CARTESIAN_POINT ( 'NONE',  ( 0.000000000000000000, 0.4692913385826771866, 0.2374015748031496065 ) ) ;
#7619=EDGE_LOOP ( 'NONE', ( #13085, #3377 ) ) ;
#7621=DIRECTION ( 'NONE',  ( 0.000000000000000000, 1.000000000000000000, 0.000000000000000000 ) ) ;
#7642=EDGE_LOOP ( 'NONE', ( #23460, #10976, #22405, #2092 ) ) ;
#7651=CARTESIAN_POINT ( 'NONE',  ( -0.3412792617076849111, 0.05967164814832635888, 0.1377952755905512139 ) ) ;
#7672=AXIS2_PLACEMENT_3D ( 'NONE', #6107, #14741, #18786 ) ;
#7682=CARTESIAN_POINT ( 'NONE',  ( -0.1285103288269285327, -0.3545966721392122545, 0.1992125984251968684 ) ) ;
#7683=ORIENTED_EDGE ( 'NONE', *, *, #14494, .T. ) ;
#7695=CARTESIAN_POINT ( 'NONE',  ( -0.2299571666338338372, 0.2748389101991166039, 0.1805249803347109272 ) ) ;
#7713=ORIENTED_EDGE ( 'NONE', *, *, #19012, .F. ) ;
#7719=EDGE_LOOP ( 'NONE', ( #19300, #2366 ) ) ;
#7722=CARTESIAN_POINT ( 'NONE',  ( -0.1599629598573824862, -0.4411872753631803090, 0.07637795275590551769 ) ) ;
#7727=DIRECTION ( 'NONE',  ( 0.8660254037844390407, -0.4999999999999994449, 0.000000000000000000 ) ) ;
#7744=CARTESIAN_POINT ( 'NONE',  ( -0.3268074212154853941, -0.1882834141668338901, 0.07637630750536809898 ) ) ;
#7748=ORIENTED_EDGE ( 'NONE', *, *, #8491, .T. ) ;
#7768=CARTESIAN_POINT ( 'NONE',  ( 0.4622285577935968948, 0.08111201067590689817, 0.1992142434433712694 ) ) ;
#7784=ORIENTED_EDGE ( 'NONE', *, *, #22572, .F. ) ;
#7787=DIMENSIONAL_EXPONENTS ( 1.000000000000000000, 0.000000000000000000, 0.000000000000000000, 0.000000000000000000, 0.000000000000000000, 0.000000000000000000, 0.000000000000000000 ) ;
#7794=EDGE_CURVE ( 'NONE', #17730, #7534, #15824, .T. ) ;
#7799=EDGE_LOOP ( 'NONE', ( #5936, #15650 ) ) ;
#7800=DIRECTION ( 'NONE',  ( 0.000000000000000000, 0.000000000000000000, 1.000000000000000000 ) ) ;
#7809=VERTEX_POINT ( 'NONE', #634 ) ;
#7815=ORIENTED_EDGE ( 'NONE', *, *, #21103, .F. ) ;
#7826=CARTESIAN_POINT ( 'NONE',  ( 0.2420394123212937232, 0.2892587550802425134, 0.07637795275590551769 ) ) ;
#7833=FACE_OUTER_BOUND ( 'NONE', #22512, .T. ) ;
#7834=EDGE_CURVE ( 'NONE', #21486, #25722, #11635, .T. ) ;
#7840=AXIS2_PLACEMENT_3D ( 'NONE', #1683, #9877, #12426 ) ;
#7847=ORIENTED_EDGE ( 'NONE', *, *, #27863, .T. ) ;
#7854=ADVANCED_FACE ( 'NONE', ( #7257 ), #22602, .F. ) ;
#7857=DIRECTION ( 'NONE',  ( 1.000000000000000000, 0.000000000000000000, 0.000000000000000000 ) ) ;
#7863=DIRECTION ( 'NONE',  ( 0.6427876096865398070, 0.7660444431189775694, -0.000000000000000000 ) ) ;
#7878=ORIENTED_EDGE ( 'NONE', *, *, #23993, .T. ) ;
#7880=CARTESIAN_POINT ( 'NONE',  ( -0.3713448905834433322, 0.06600512665679449109, 0.1992125984251968684 ) ) ;
#7913=EDGE_CURVE ( 'NONE', #3462, #21723, #18046, .T. ) ;
#7923=DIRECTION ( 'NONE',  ( 1.000000000000000000, 0.000000000000000000, 0.000000000000000000 ) ) ;
#7924=CARTESIAN_POINT ( 'NONE',  ( 0.1291602287245497971, -0.3543605079199910191, 0.07637549214372835182 ) ) ;
#7927=CARTESIAN_POINT ( 'NONE',  ( 0.3012109481301854519, 0.3598698725862389813, 0.1992125984251968684 ) ) ;
#7931=FACE_BOUND ( 'NONE', #18262, .T. ) ;
#7945=CARTESIAN_POINT ( 'NONE',  ( 0.000000000000000000, 0.000000000000000000, 0.1377952755905511861 ) ) ;
#7958=AXIS2_PLACEMENT_3D ( 'NONE', #21654, #8783, #343 ) ;
#7968=CARTESIAN_POINT ( 'NONE',  ( 0.000000000000000000, 0.5511811023622047445, 0.1377952755905511861 ) ) ;
#7984=ORIENTED_EDGE ( 'NONE', *, *, #7491, .F. ) ;
#7997=CARTESIAN_POINT ( 'NONE',  ( 0.3012109481301854519, 0.3598698725862389813, 0.1992125984251968684 ) ) ;
#8010=CARTESIAN_POINT ( 'NONE',  ( 0.4167985568850881561, 0.07349283109919291235, 0.1377952755905511861 ) ) ;
#8016=CARTESIAN_POINT ( 'NONE',  ( 0.3012109481302311376, 0.3598698725862007897, 0.07637795275590551769 ) ) ;
#8022=ADVANCED_FACE ( 'NONE', ( #14334, #7833 ), #12063, .T. ) ;
#8023=VERTEX_POINT ( 'NONE', #9799 ) ;
#8040=B_SPLINE_CURVE_WITH_KNOTS ( 'NONE', 3,
 ( #17615, #2354, #21997, #10986, #4613, #21862 ),
 .UNSPECIFIED., .F., .F.,
 ( 4, 2, 4 ),
 ( 0.6902184472752670441, 0.6915327610580710438, 0.6928470748408740443 ),
 .UNSPECIFIED. ) ;
#8043=ORIENTED_EDGE ( 'NONE', *, *, #4386, .F. ) ;
#8046=ORIENTED_EDGE ( 'NONE', *, *, #1431, .T. ) ;
#8050=CARTESIAN_POINT ( 'NONE',  ( -0.3607825703597850042, 0.06309631803674747852, 0.1910323753036148042 ) ) ;
#8054=ORIENTED_EDGE ( 'NONE', *, *, #8607, .F. ) ;
#8065=CARTESIAN_POINT ( 'NONE',  ( 0.2428345617565153547, 0.2885915454824177218, 0.1992125984251968684 ) ) ;
#8069=VERTEX_POINT ( 'NONE', #24910 ) ;
#8089=FACE_OUTER_BOUND ( 'NONE', #1848, .T. ) ;
#8093=DIRECTION ( 'NONE',  ( 0.000000000000000000, -1.000000000000000000, 0.000000000000000000 ) ) ;
#8101=COLOUR_RGB ( '', 0.08235294, 0.09019608, 0.10196078) ;
#8114=AXIS2_PLACEMENT_3D ( 'NONE', #128, #6315, #8698 ) ;
#8116=EDGE_CURVE ( 'NONE', #1085, #14294, #23818, .T. ) ;
#8124=VERTEX_POINT ( 'NONE', #4656 ) ;
#8145=CARTESIAN_POINT ( 'NONE',  ( -1.456051859514965975E-17, 0.4692913385826771866, 0.1992150590373740204 ) ) ;
#8157=CARTESIAN_POINT ( 'NONE',  ( 0.3209354104558860277, 0.3834063931588274077, 0.1496602734615972985 ) ) ;
#8164=DIRECTION ( 'NONE',  ( 1.000000000000000000, 0.000000000000000000, 0.000000000000000000 ) ) ;
#8167=CARTESIAN_POINT ( 'NONE',  ( -0.3015429802557554329, -0.1746717017760298918, 0.1166443193911902154 ) ) ;
#8173=CARTESIAN_POINT ( 'NONE',  ( -0.1658689444494333143, -0.4574452598450142737, 0.09284957166512360083 ) ) ;
#8181=EDGE_CURVE ( 'NONE', #24304, #6563, #17653, .T. ) ;
#8184=CARTESIAN_POINT ( 'NONE',  ( -0.3529960615022087467, 0.06172929298840394013, 0.1805249803415331367 ) ) ;
#8190=EDGE_CURVE ( 'NONE', #8124, #14678, #9076, .T. ) ;
#8196=CARTESIAN_POINT ( 'NONE',  ( -0.4621951630817676682, 0.08130208312401832060, 0.07637549214372854611 ) ) ;
#8204=CARTESIAN_POINT ( 'NONE',  ( 0.4232283464566928832, 0.000000000000000000, 0.1377952755905511861 ) ) ;
#8212=CARTESIAN_POINT ( 'NONE',  ( 0.2420394123212937232, 0.2892587550802425134, 0.07637795275590551769 ) ) ;
#8217=CARTESIAN_POINT ( 'NONE',  ( -0.0005789221761214173069, 0.4692909815006417462, 0.07637795275590551769 ) ) ;
#8228=CARTESIAN_POINT ( 'NONE',  ( 0.5393700787401575214, 0.000000000000000000, 0.2637795275590551491 ) ) ;
#8235=ORIENTED_EDGE ( 'NONE', *, *, #9210, .T. ) ;
#8238=ORIENTED_EDGE ( 'NONE', *, *, #22758, .T. ) ;
#8240=CARTESIAN_POINT ( 'NONE',  ( -0.3715251363271980245, 0.06498290224717540031, 0.07637795275590551769 ) ) ;
#8253=EDGE_LOOP ( 'NONE', ( #8318, #21304 ) ) ;
#8283=CARTESIAN_POINT ( 'NONE',  ( 0.4066108233583488052, -0.2343118354750409471, 0.1992142434433716580 ) ) ;
#8286=B_SPLINE_CURVE_WITH_KNOTS ( 'NONE', 3,
 ( #15969, #24571, #24994, #22893, #12011, #14578 ),
 .UNSPECIFIED., .F., .F.,
 ( 4, 2, 4 ),
 ( 0.7157687286427130147, 0.7172350147555660582, 0.7187013008684189908 ),
 .UNSPECIFIED. ) ;
#8295=DIRECTION ( 'NONE',  ( 0.000000000000000000, 0.000000000000000000, 1.000000000000000000 ) ) ;
#8300=CARTESIAN_POINT ( 'NONE',  ( 0.000000000000000000, 0.000000000000000000, 0.01181102362204724393 ) ) ;
#8315=CARTESIAN_POINT ( 'NONE',  ( -0.1694923354741917354, -0.4674199084399158766, 0.1615162260944750239 ) ) ;
#8316=CIRCLE ( 'NONE', #27716, 0.01181102362204724046 ) ;
#8318=ORIENTED_EDGE ( 'NONE', *, *, #18492, .F. ) ;
#8328=AXIS2_PLACEMENT_3D ( 'NONE', #3705, #15811, #7621 ) ;
#8350=CARTESIAN_POINT ( 'NONE',  ( 0.1288360683667812978, -0.3544784926413476200, 0.07637549214372835182 ) ) ;
#8360=CARTESIAN_POINT ( 'NONE',  ( -0.0005847768872542869270, 0.4787829797961313250, 0.08349695147752332625 ) ) ;
#8368=ORIENTED_EDGE ( 'NONE', *, *, #4204, .T. ) ;
#8374=CARTESIAN_POINT ( 'NONE',  ( 0.000000000000000000, 0.4232283464566928832, -3.341531889763779686E-17 ) ) ;
#8387=ORIENTED_EDGE ( 'NONE', *, *, #8190, .T. ) ;
#8389=TOROIDAL_SURFACE ( 'NONE', #13796, 0.4232283464566928832, 0.07677165354330708902 ) ;
#8391=LINE ( 'NONE', #7968, #11283 ) ;
#8392=CARTESIAN_POINT ( 'NONE',  ( -0.3715251363271980245, 0.06498290224717540031, 0.07637795275590551769 ) ) ;
#8393=CARTESIAN_POINT ( 'NONE',  ( 0.1658689444493339771, -0.4574452598447248941, 0.09284957166472920798 ) ) ;
#8414=ORIENTED_EDGE ( 'NONE', *, *, #4633, .T. ) ;
#8430=DIRECTION ( 'NONE',  ( 0.000000000000000000, 0.000000000000000000, 1.000000000000000000 ) ) ;
#8435=DIRECTION ( 'NONE',  ( 0.000000000000000000, 0.000000000000000000, 1.000000000000000000 ) ) ;
#8439=ORIENTED_EDGE ( 'NONE', *, *, #2323, .T. ) ;
#8445=ORIENTED_EDGE ( 'NONE', *, *, #27546, .F. ) ;
#8474=AXIS2_PLACEMENT_3D ( 'NONE', #3004, #9226, #9368 ) ;
#8475=CARTESIAN_POINT ( 'NONE',  ( 0.3267210193396165585, -0.1884333032645078565, 0.07637549214372835182 ) ) ;
#8486=CARTESIAN_POINT ( 'NONE',  ( 0.000000000000000000, 0.000000000000000000, 0.1992125984251968684 ) ) ;
#8488=CARTESIAN_POINT ( 'NONE',  ( 0.000000000000000000, 0.000000000000000000, 0.03818897637795275884 ) ) ;
#8491=EDGE_CURVE ( 'NONE', #21339, #19933, #6128, .T. ) ;
#8496=FACE_OUTER_BOUND ( 'NONE', #22266, .T. ) ;
#8503=CARTESIAN_POINT ( 'NONE',  ( 0.1606879121748897576, -0.4409237942971110380, 0.07637549214372854611 ) ) ;
#8522=DIRECTION ( 'NONE',  ( -0.6427876096865396960, -0.7660444431189776804, 0.000000000000000000 ) ) ;
#8530=AXIS2_PLACEMENT_3D ( 'NONE', #14081, #12521, #3466 ) ;
#8563=CARTESIAN_POINT ( 'NONE',  ( 0.3263749705684267921, -0.1890319631540330891, 0.1992125984251968684 ) ) ;
#8567=CIRCLE ( 'NONE', #6779, 0.4692913385826771866 ) ;
#8578=VERTEX_POINT ( 'NONE', #13312 ) ;
#8607=EDGE_CURVE ( 'NONE', #14590, #26957, #3676, .T. ) ;
#8610=ORIENTED_EDGE ( 'NONE', *, *, #13706, .F. ) ;
#8624=ORIENTED_EDGE ( 'NONE', *, *, #20229, .F. ) ;
#8642=ORIENTED_EDGE ( 'NONE', *, *, #11446, .T. ) ;
#8643=EDGE_CURVE ( 'NONE', #23407, #7809, #11363, .T. ) ;
#8655=PRESENTATION_STYLE_ASSIGNMENT (( #222 ) ) ;
#8672=EDGE_CURVE ( 'NONE', #8578, #2204, #18903, .T. ) ;
#8675=DIRECTION ( 'NONE',  ( 0.000000000000000000, 0.000000000000000000, 1.000000000000000000 ) ) ;
#8677=B_SPLINE_CURVE_WITH_KNOTS ( 'NONE', 3,
 ( #8145, #25365, #1913, #25511 ),
 .UNSPECIFIED., .F., .F.,
 ( 4, 4 ),
 ( 0.7172350147555668354, 0.7187013008684189908 ),
 .UNSPECIFIED. ) ;
#8682=CARTESIAN_POINT ( 'NONE',  ( -0.3018020646414484309, 0.3593743330771480560, 0.1992150590373740204 ) ) ;
#8689=CARTESIAN_POINT ( 'NONE',  ( 0.2421724791772047192, 0.2891474103999575052, 0.07637630750536809898 ) ) ;
#8698=DIRECTION ( 'NONE',  ( 0.000000000000000000, -1.000000000000000000, 0.000000000000000000 ) ) ;
#8699=ORIENTED_EDGE ( 'NONE', *, *, #5118, .F. ) ;
#8705=ORIENTED_EDGE ( 'NONE', *, *, #1983, .F. ) ;
#8712=CYLINDRICAL_SURFACE ( 'NONE', #19015, 0.3771653543307086909 ) ;
#8715=VERTEX_POINT ( 'NONE', #20926 ) ;
#8731=TOROIDAL_SURFACE ( 'NONE', #12330, 0.5393700787401575214, 0.01181102362204724393 ) ;
#8753=ORIENTED_EDGE ( 'NONE', *, *, #7834, .F. ) ;
#8762=CARTESIAN_POINT ( 'NONE',  ( 0.5511811023622047445, 0.000000000000000000, 0.2637795275590551491 ) ) ;
#8768=DIRECTION ( 'NONE',  ( 0.4999999999999994449, -0.8660254037844389297, 0.000000000000000000 ) ) ;
#8769=CARTESIAN_POINT ( 'NONE',  ( 0.000000000000000000, 0.000000000000000000, 0.07637795275590551769 ) ) ;
#8774=AXIS2_PLACEMENT_3D ( 'NONE', #27452, #14623, #18961 ) ;
#8783=DIRECTION ( 'NONE',  ( 0.000000000000000000, 0.000000000000000000, 1.000000000000000000 ) ) ;
#8785=CARTESIAN_POINT ( 'NONE',  ( -0.2230788859036006710, 0.2650812153444457864, 0.1478915661164160456 ) ) ;
#8791=FACE_OUTER_BOUND ( 'NONE', #7642, .T. ) ;
#8792=DIRECTION ( 'NONE',  ( 0.7660444431189777914, -0.6427876096865395850, 0.000000000000000000 ) ) ;
#8803=AXIS2_PLACEMENT_3D ( 'NONE', #24673, #18591, #18308 ) ;
#8816=CARTESIAN_POINT ( 'NONE',  ( 0.000000000000000000, 0.000000000000000000, 0.03818897637795275884 ) ) ;
#8820=ORIENTED_EDGE ( 'NONE', *, *, #5893, .F. ) ;
#8830=AXIS2_PLACEMENT_3D ( 'NONE', #15168, #26025, #2153 ) ;
#8836=CARTESIAN_POINT ( 'NONE',  ( 0.000000000000000000, 0.000000000000000000, -3.278217716535432842E-17 ) ) ;
#8839=ORIENTED_EDGE ( 'NONE', *, *, #2085, .F. ) ;
#8842=PRODUCT_CONTEXT ( 'NONE', #19006, 'mechanical' ) ;
#8846=VERTEX_POINT ( 'NONE', #27284 ) ;
#8855=ORIENTED_EDGE ( 'NONE', *, *, #8116, .F. ) ;
#8859=VERTEX_POINT ( 'NONE', #4393 ) ;
#8860=VERTEX_POINT ( 'NONE', #21769 ) ;
#8867=VERTEX_POINT ( 'NONE', #17385 ) ;
#8871=CARTESIAN_POINT ( 'NONE',  ( 0.3174445073404819628, -0.1826860508837442609, 0.1910323753066165142 ) ) ;
#8874=AXIS2_PLACEMENT_3D ( 'NONE', #19907, #13127, #22027 ) ;
#8879=CARTESIAN_POINT ( 'NONE',  ( -0.0005789221761214173069, 0.4692909815006417462, 0.07637795275590551769 ) ) ;
#8886=CARTESIAN_POINT ( 'NONE',  ( -0.4062254136079394562, -0.2349793847444822670, 0.07637630773773071424 ) ) ;
#8901=EDGE_CURVE ( 'NONE', #6630, #17458, #20378, .T. ) ;
#8902=FACE_BOUND ( 'NONE', #26860, .T. ) ;
#8921=CARTESIAN_POINT ( 'NONE',  ( 0.3430989538749588119, 0.06100393589356664648, 0.1166443193823661489 ) ) ;
#8935=AXIS2_PLACEMENT_3D ( 'NONE', #3102, #11316, #20357 ) ;
#8945=CARTESIAN_POINT ( 'NONE',  ( -0.4922996667774039437, 0.08741303158498453518, 0.1259302777225530801 ) ) ;
#8950=ADVANCED_FACE ( 'NONE', ( #6795, #10887 ), #21351, .T. ) ;
#8953=ORIENTED_EDGE ( 'NONE', *, *, #22840, .F. ) ;
#8966=CARTESIAN_POINT ( 'NONE',  ( -0.2428345617565149384, 0.2885915454824177218, 0.07637795275590551769 ) ) ;
#8976=DIRECTION ( 'NONE',  ( 0.000000000000000000, 1.000000000000000000, 0.000000000000000000 ) ) ;
#8983=AXIS2_PLACEMENT_3D ( 'NONE', #12532, #18739, #27094 ) ;
#8984=ORIENTED_EDGE ( 'NONE', *, *, #17167, .F. ) ;
#8985=DIRECTION ( 'NONE',  ( 0.000000000000000000, -1.000000000000000000, 0.000000000000000000 ) ) ;
#8987=ADVANCED_FACE ( 'NONE', ( #25729 ), #23597, .F. ) ;
#8994=ADVANCED_FACE ( 'NONE', ( #25866 ), #22451, .T. ) ;
#8997=EDGE_LOOP ( 'NONE', ( #10401, #23349, #11388, #20610, #26136 ) ) ;
#9008=FACE_BOUND ( 'NONE', #9791, .T. ) ;
#9014=CARTESIAN_POINT ( 'NONE',  ( 0.4143458349581316535, -0.2398979215371937757, 0.08349695147638480641 ) ) ;
#9015=VERTEX_POINT ( 'NONE', #26825 ) ;
#9023=CARTESIAN_POINT ( 'NONE',  ( -0.3606049308155347410, 0.06410376196632514012, 0.08455817587594735563 ) ) ;
#9036=EDGE_CURVE ( 'NONE', #21231, #1085, #5978, .T. ) ;
#9037=CARTESIAN_POINT ( 'NONE',  ( -0.0004974201395674843510, 0.3464563358313494934, 0.1478915661211720467 ) ) ;
#9038=CARTESIAN_POINT ( 'NONE',  ( 0.4620608682196457040, 0.08206165078054626638, 0.07637795275590551769 ) ) ;
#9040=CARTESIAN_POINT ( 'NONE',  ( -0.2425693455392318731, 0.2888145544500153594, 0.07637549214372854611 ) ) ;
#9041=ORIENTED_EDGE ( 'NONE', *, *, #6155, .T. ) ;
#9043=CARTESIAN_POINT ( 'NONE',  ( -0.3218517393633636980, 0.3826375019116435294, 0.1259302777250448369 ) ) ;
#9067=DIRECTION ( 'NONE',  ( 0.000000000000000000, 0.000000000000000000, 1.000000000000000000 ) ) ;
#9073=CARTESIAN_POINT ( 'NONE',  ( 0.000000000000000000, 0.000000000000000000, 0.1377952755905511861 ) ) ;
#9074=CARTESIAN_POINT ( 'NONE',  ( 0.3200513472073915344, 0.3804946224884545591, 0.1615162260904031422 ) ) ;
#9076=CIRCLE ( 'NONE', #19010, 0.4692913385826771866 ) ;
#9102=SPHERICAL_SURFACE ( 'NONE', #16835, 0.07677362204724409722 ) ;
#9104=ORIENTED_EDGE ( 'NONE', *, *, #24328, .F. ) ;
#9110=B_SPLINE_CURVE_WITH_KNOTS ( 'NONE', 3,
 ( #25935, #385, #2601, #4326, #6728, #8966 ),
 .UNSPECIFIED., .F., .F.,
 ( 4, 2, 4 ),
 ( 0.5000000000000000000, 0.7500000000000000000, 1.000000000000000000 ),
 .UNSPECIFIED. ) ;
#9131=ORIENTED_EDGE ( 'NONE', *, *, #25291, .F. ) ;
#9152=ORIENTED_EDGE ( 'NONE', *, *, #26098, .T. ) ;
#9153=ORIENTED_EDGE ( 'NONE', *, *, #355, .T. ) ;
#9160=CARTESIAN_POINT ( 'NONE',  ( 0.000000000000000000, 0.000000000000000000, 0.1992125984251968684 ) ) ;
#9161=CARTESIAN_POINT ( 'NONE',  ( 0.1257482708759803669, -0.3439950301957984680, 0.08455817587492829579 ) ) ;
#9174=DIRECTION ( 'NONE',  ( 0.000000000000000000, 1.000000000000000000, 0.000000000000000000 ) ) ;
#9177=AXIS2_PLACEMENT_3D ( 'NONE', #13385, #4508, #13115 ) ;
#9181=ORIENTED_EDGE ( 'NONE', *, *, #23103, .F. ) ;
#9198=CARTESIAN_POINT ( 'NONE',  ( -0.4211031283167419592, -0.2438048970097803081, 0.1827409795204104903 ) ) ;
#9202=CARTESIAN_POINT ( 'NONE',  ( 0.000000000000000000, 0.000000000000000000, 0.2637795275590551491 ) ) ;
#9210=EDGE_CURVE ( 'NONE', #10703, #5544, #15462, .T. ) ;
#9211=CIRCLE ( 'NONE', #3814, 0.3771653543307086909 ) ;
#9222=DIRECTION ( 'NONE',  ( 1.000000000000000000, 0.000000000000000000, 0.000000000000000000 ) ) ;
#9226=DIRECTION ( 'NONE',  ( 0.000000000000000000, 0.000000000000000000, 1.000000000000000000 ) ) ;
#9238=DIMENSIONAL_EXPONENTS ( 1.000000000000000000, 0.000000000000000000, 0.000000000000000000, 0.000000000000000000, 0.000000000000000000, 0.000000000000000000, 0.000000000000000000 ) ;
#9240=DIRECTION ( 'NONE',  ( 0.000000000000000000, 0.000000000000000000, -1.000000000000000000 ) ) ;
#9249=VERTEX_POINT ( 'NONE', #3217 ) ;
#9260=DIRECTION ( 'NONE',  ( 0.000000000000000000, -1.000000000000000000, 0.000000000000000000 ) ) ;
#9266=DIRECTION ( 'NONE',  ( 0.000000000000000000, 1.000000000000000000, 0.000000000000000000 ) ) ;
#9280=CARTESIAN_POINT ( 'NONE',  ( -0.4925073816770652591, 0.08623502184940523563, 0.1496602734601975015 ) ) ;
#9281=EDGE_CURVE ( 'NONE', #25040, #20898, #182, .T. ) ;
#9287=ORIENTED_EDGE ( 'NONE', *, *, #21474, .F. ) ;
#9292=EDGE_CURVE ( 'NONE', #12348, #14826, #17508, .T. ) ;
#9306=CARTESIAN_POINT ( 'NONE',  ( 0.000000000000000000, 0.000000000000000000, 0.1377952755905511861 ) ) ;
#9368=DIRECTION ( 'NONE',  ( 0.000000000000000000, 1.000000000000000000, 0.000000000000000000 ) ) ;
#9372=TOROIDAL_SURFACE ( 'NONE', #23856, 0.4232283464566928832, 0.07677165354330708902 ) ;
#9383=DIRECTION ( 'NONE',  ( 0.000000000000000000, 0.000000000000000000, 1.000000000000000000 ) ) ;
#9395=ORIENTED_EDGE ( 'NONE', *, *, #25615, .T. ) ;
#9397=SPHERICAL_SURFACE ( 'NONE', #9469, 0.07677362204724409722 ) ;
#9409=DIRECTION ( 'NONE',  ( 0.1736481776669309696, 0.9848077530122079093, 0.000000000000000000 ) ) ;
#9411=TOROIDAL_SURFACE ( 'NONE', #8983, 0.4232283464566928832, 0.07677165354330708902 ) ;
#9422=CARTESIAN_POINT ( 'NONE',  ( 0.3263749705684267921, -0.1890319631540330891, 0.07637795275590551769 ) ) ;
#9423=EDGE_LOOP ( 'NONE', ( #11393, #10472 ) ) ;
#9447=CARTESIAN_POINT ( 'NONE',  ( -0.3123213164510841300, 0.3731274149342653224, 0.09284957166224125369 ) ) ;
#9450=CYLINDRICAL_SURFACE ( 'NONE', #9663, 0.5511811023622047445 ) ;
#9451=CARTESIAN_POINT ( 'NONE',  ( 0.000000000000000000, 0.000000000000000000, 0.07637795275590551769 ) ) ;
#9458=EDGE_CURVE ( 'NONE', #21231, #5544, #22380, .T. ) ;
#9466=ORIENTED_EDGE ( 'NONE', *, *, #18141, .F. ) ;
#9469=AXIS2_PLACEMENT_3D ( 'NONE', #2636, #5316, #5032 ) ;
#9477=AXIS2_PLACEMENT_3D ( 'NONE', #27498, #7863, #10105 ) ;
#9481=CARTESIAN_POINT ( 'NONE',  ( 0.3714653163189441387, 0.06532421472592657430, 0.1992150590373740204 ) ) ;
#9493=DIRECTION ( 'NONE',  ( 0.000000000000000000, 0.000000000000000000, 1.000000000000000000 ) ) ;
#9499=CARTESIAN_POINT ( 'NONE',  ( 0.4067073728345488304, -0.2341441294389854655, 0.07637795275590551769 ) ) ;
#9500=CARTESIAN_POINT ( 'NONE',  ( 0.3713448905834433322, 0.06600512665679410251, 0.07637795275590551769 ) ) ;
#9503=DIRECTION ( 'NONE',  ( 0.000000000000000000, 0.000000000000000000, 1.000000000000000000 ) ) ;
#9508=B_SPLINE_CURVE_WITH_KNOTS ( 'NONE', 3,
 ( #15122, #8871, #12836, #12693, #420, #19336 ),
 .UNSPECIFIED., .F., .F.,
 ( 4, 2, 4 ),
 ( 0.000000000000000000, 0.2500000000000001665, 0.5000000000000000000 ),
 .UNSPECIFIED. ) ;
#9523=CARTESIAN_POINT ( 'NONE',  ( 0.3529960615022520454, 0.06172929298841274559, 0.1805249803415999998 ) ) ;
#9534=ORIENTED_EDGE ( 'NONE', *, *, #23489, .F. ) ;
#9546=CARTESIAN_POINT ( 'NONE',  ( -0.4065144339881338054, -0.2344790234878023627, 0.1992150590373740204 ) ) ;
#9569=VERTEX_POINT ( 'NONE', #16878 ) ;
#9578=CARTESIAN_POINT ( 'NONE',  ( -0.4620947063919622066, 0.08187111969652559329, 0.1992142434433716580 ) ) ;
#9579=DIRECTION ( 'NONE',  ( 0.000000000000000000, 1.000000000000000000, 0.000000000000000000 ) ) ;
#9609=( CONVERSION_BASED_UNIT ( 'INCH', #6823 ) LENGTH_UNIT ( ) NAMED_UNIT ( #7787 ) ) ;
#9612=AXIS2_PLACEMENT_3D ( 'NONE', #24329, #4977, #19439 ) ;
#9613=CIRCLE ( 'NONE', #1006, 0.07677362204724411110 ) ;
#9616=ADVANCED_FACE ( 'NONE', ( #4017 ), #6151, .F. ) ;
#9617=EDGE_LOOP ( 'NONE', ( #13184, #26695, #14076, #18493 ) ) ;
#9621=CARTESIAN_POINT ( 'NONE',  ( -0.3714054139060130044, 0.06566393819133267695, 0.07637549214372835182 ) ) ;
#9640=CARTESIAN_POINT ( 'NONE',  ( 6.557635703933409897E-17, 0.3771653543307084688, 0.07637549214372833795 ) ) ;
#9649=CARTESIAN_POINT ( 'NONE',  ( -0.1610509776512594748, -0.4407912692718567449, 0.1992125984251968684 ) ) ;
#9658=ORIENTED_EDGE ( 'NONE', *, *, #11931, .T. ) ;
#9663=AXIS2_PLACEMENT_3D ( 'NONE', #18050, #7350, #9174 ) ;
#9670=CIRCLE ( 'NONE', #27748, 0.01181102362204724393 ) ;
#9672=FACE_OUTER_BOUND ( 'NONE', #25485, .T. ) ;
#9682=ORIENTED_EDGE ( 'NONE', *, *, #11287, .F. ) ;
#9686=ORIENTED_EDGE ( 'NONE', *, *, #13053, .F. ) ;
#9690=FACE_BOUND ( 'NONE', #13395, .T. ) ;
#9695=CARTESIAN_POINT ( 'NONE',  ( 0.000000000000000000, 0.4232283464566928832, 0.1377952755905511861 ) ) ;
#9704=ORIENTED_EDGE ( 'NONE', *, *, #235, .F. ) ;
#9706=CARTESIAN_POINT ( 'NONE',  ( -0.5511811023622047445, 6.750021727583836750E-17, 0.01181102362204724393 ) ) ;
#9719=CARTESIAN_POINT ( 'NONE',  ( 0.2997912780622379869, -0.1736589463928938648, 0.1276989850557191386 ) ) ;
#9720=VERTEX_POINT ( 'NONE', #23237 ) ;
#9731=DIRECTION ( 'NONE',  ( 0.000000000000000000, 0.000000000000000000, -1.000000000000000000 ) ) ;
#9749=EDGE_LOOP ( 'NONE', ( #23816, #1511, #13817, #25074, #6867 ) ) ;
#9761=CARTESIAN_POINT ( 'NONE',  ( 0.1220886091262543827, -0.3369140789136257363, 0.1805249803408568721 ) ) ;
#9763=ORIENTED_EDGE ( 'NONE', *, *, #2035, .F. ) ;
#9765=ORIENTED_EDGE ( 'NONE', *, *, #18798, .F. ) ;
#9777=ADVANCED_FACE ( 'NONE', ( #6688 ), #19087, .F. ) ;
#9791=EDGE_LOOP ( 'NONE', ( #16749, #23485, #24091, #27621 ) ) ;
#9793=VERTEX_POINT ( 'NONE', #2435 ) ;
#9799=CARTESIAN_POINT ( 'NONE',  ( 0.3070866141732283561, 0.000000000000000000, 0.2755905511811023723 ) ) ;
#9800=ORIENTED_EDGE ( 'NONE', *, *, #16746, .F. ) ;
#9805=APPLICATION_CONTEXT ( 'automotive_design' ) ;
#9819=VERTEX_POINT ( 'NONE', #226 ) ;
#9842=AXIS2_PLACEMENT_3D ( 'NONE', #24753, #16008, #26877 ) ;
#9852=VECTOR ( 'NONE', #12379, 39.37007874015748143 ) ;
#9873=CARTESIAN_POINT ( 'NONE',  ( 0.4621951630817700551, 0.08130208312399862802, 0.1992150590373740204 ) ) ;
#9877=DIRECTION ( 'NONE',  ( 0.000000000000000000, 0.000000000000000000, 1.000000000000000000 ) ) ;
#9879=UNCERTAINTY_MEASURE_WITH_UNIT (LENGTH_MEASURE( 1.000000000000000082E-05 ), #9609, 'distance_accuracy_value', 'NONE') ;
#9882=CARTESIAN_POINT ( 'NONE',  ( 0.4061284506584276199, -0.2351468520616558922, 0.07637795275590551769 ) ) ;
#9930=CARTESIAN_POINT ( 'NONE',  ( -0.4216927985375814592, -0.2427835582314765150, 0.09284957166320603750 ) ) ;
#9934=CARTESIAN_POINT ( 'NONE',  ( 0.3715251363271980245, 0.06498290224717499786, 0.07637795275590551769 ) ) ;
#9950=ORIENTED_EDGE ( 'NONE', *, *, #21075, .F. ) ;
#9962=CARTESIAN_POINT ( 'NONE',  ( 0.1285103288269283661, -0.3545966721392122545, 0.1992125984251968684 ) ) ;
#9984=CARTESIAN_POINT ( 'NONE',  ( -0.3020979083623086536, 0.3591256245825952265, 0.07637795275590551769 ) ) ;
#9996=AXIS2_PLACEMENT_3D ( 'NONE', #10633, #19256, #4014 ) ;
#10011=B_SPLINE_CURVE_WITH_KNOTS ( 'NONE', 3,
 ( #4853, #8689, #2725, #15355, #11358, #15203 ),
 .UNSPECIFIED., .F., .F.,
 ( 4, 2, 4 ),
 ( 0.2291966065698859967, 0.2305109203526899964, 0.2318252341354939960 ),
 .UNSPECIFIED. ) ;
#10012=CARTESIAN_POINT ( 'NONE',  ( -0.3432721300517010965, 0.06002180498082090171, 0.1589462317926021162 ) ) ;
#10013=EDGE_CURVE ( 'NONE', #5387, #27620, #3763, .T. ) ;
#10014=CARTESIAN_POINT ( 'NONE',  ( 0.4620947063919622066, 0.08187111969652538512, 0.1992142434433712694 ) ) ;
#10015=CARTESIAN_POINT ( 'NONE',  ( -0.4620608682196346573, 0.08206165078060512208, 0.1992125984251968684 ) ) ;
#10035=DIRECTION ( 'NONE',  ( 1.000000000000000000, 0.000000000000000000, 0.000000000000000000 ) ) ;
#10040=CARTESIAN_POINT ( 'NONE',  ( -0.0005847768872418040737, 0.4787829797941598464, 0.1920935997050576827 ) ) ;
#10105=DIRECTION ( 'NONE',  ( -0.7660444431189775694, 0.6427876096865401401, 0.000000000000000000 ) ) ;
#10122=ORIENTED_EDGE ( 'NONE', *, *, #5150, .F. ) ;
#10132=EDGE_CURVE ( 'NONE', #1951, #5345, #15063, .T. ) ;
#10145=DIRECTION ( 'NONE',  ( 0.000000000000000000, 1.000000000000000000, 0.000000000000000000 ) ) ;
#10151=CARTESIAN_POINT ( 'NONE',  ( -0.1447526197146041249, -0.3977045540727763839, 0.2145688976377952695 ) ) ;
#10158=ORIENTED_EDGE ( 'NONE', *, *, #19573, .T. ) ;
#10162=ORIENTED_EDGE ( 'NONE', *, *, #9292, .T. ) ;
#10170=CIRCLE ( 'NONE', #23299, 0.4692913385826771866 ) ;
#10249=TOROIDAL_SURFACE ( 'NONE', #26048, 0.4232283464566928832, 0.07677165354330708902 ) ;
#10252=CARTESIAN_POINT ( 'NONE',  ( 0.3209354104564642318, 0.3834063931595186880, 0.1259302777253356043 ) ) ;
#10262=CARTESIAN_POINT ( 'NONE',  ( 0.000000000000000000, 0.2952755905511810774, 0.2637795275590551491 ) ) ;
#10263=CARTESIAN_POINT ( 'NONE',  ( -0.3169330146478837040, -0.1835719822040729754, 0.08455817587859276729 ) ) ;
#10277=VERTEX_POINT ( 'NONE', #23048 ) ;
#10279=CARTESIAN_POINT ( 'NONE',  ( -0.3715251363271980245, 0.06498290224717540031, 0.1992125984251968684 ) ) ;
#10285=CARTESIAN_POINT ( 'NONE',  ( 0.000000000000000000, 0.000000000000000000, 0.2637795275590551491 ) ) ;
#10288=FACE_BOUND ( 'NONE', #6924, .T. ) ;
#10295=CARTESIAN_POINT ( 'NONE',  ( 0.3070866141732283561, 0.000000000000000000, -1.639108858267716421E-17 ) ) ;
#10297=TOROIDAL_SURFACE ( 'NONE', #12119, 0.4232283464566928832, 0.07677165354330708902 ) ;
#10303=ORIENTED_EDGE ( 'NONE', *, *, #17167, .T. ) ;
#10336=DIRECTION ( 'NONE',  ( 0.000000000000000000, 0.000000000000000000, 1.000000000000000000 ) ) ;
#10346=CARTESIAN_POINT ( 'NONE',  ( -0.1285103288269285327, -0.3545966721392122545, 0.1992125984251968684 ) ) ;
#10352=DIRECTION ( 'NONE',  ( 0.000000000000000000, 0.000000000000000000, 1.000000000000000000 ) ) ;
#10354=CARTESIAN_POINT ( 'NONE',  ( 0.1658689444481890873, -0.4574452598415587601, 0.1827409795207127485 ) ) ;
#10357=EDGE_CURVE ( 'NONE', #17040, #3411, #17791, .T. ) ;
#10366=VERTEX_POINT ( 'NONE', #27107 ) ;
#10367=VERTEX_POINT ( 'NONE', #16368 ) ;
#10372=CIRCLE ( 'NONE', #3139, 0.07677362204724411110 ) ;
#10376=DIRECTION ( 'NONE',  ( 0.000000000000000000, 0.000000000000000000, 1.000000000000000000 ) ) ;
#10384=CARTESIAN_POINT ( 'NONE',  ( 0.4062254136079196942, -0.2349793847445169337, 0.1992142434433712694 ) ) ;
#10388=VERTEX_POINT ( 'NONE', #27530 ) ;
#10391=EDGE_CURVE ( 'NONE', #15450, #13929, #9613, .T. ) ;
#10397=ADVANCED_FACE ( 'NONE', ( #18318 ), #27632, .T. ) ;
#10399=CIRCLE ( 'NONE', #13106, 0.07677362204724411110 ) ;
#10401=ORIENTED_EDGE ( 'NONE', *, *, #6361, .T. ) ;
#10403=CARTESIAN_POINT ( 'NONE',  ( 0.000000000000000000, 0.000000000000000000, 0.2637795275590551491 ) ) ;
#10432=ADVANCED_FACE ( 'NONE', ( #15236 ), #19496, .F. ) ;
#10435=B_SPLINE_CURVE_WITH_KNOTS ( 'NONE', 3,
 ( #3872, #16882, #25626, #6280, #19262, #6691, #604, #9198, #21529, #2439 ),
 .UNSPECIFIED., .F., .F.,
 ( 4, 2, 2, 2, 4 ),
 ( 0.000000000000000000, 0.2500000000000000000, 0.5000000000000000000, 0.7500000000000000000, 1.000000000000000000 ),
 .UNSPECIFIED. ) ;
#10447=ORIENTED_EDGE ( 'NONE', *, *, #11304, .T. ) ;
#10455=CARTESIAN_POINT ( 'NONE',  ( -0.3606049308151464960, 0.06410376196625482137, 0.1910323753048591700 ) ) ;
#10460=CARTESIAN_POINT ( 'NONE',  ( 0.000000000000000000, 0.4232283464566928832, 0.2755905511811023723 ) ) ;
#10472=ORIENTED_EDGE ( 'NONE', *, *, #27640, .T. ) ;
#10477=ORIENTED_EDGE ( 'NONE', *, *, #16975, .F. ) ;
#10491=CARTESIAN_POINT ( 'NONE',  ( 0.1704479274145334344, -0.4700505334969884430, 0.1259302777270377427 ) ) ;
#10494=CARTESIAN_POINT ( 'NONE',  ( 0.3713448905834433322, 0.06600512665679410251, 0.1992125984251968684 ) ) ;
#10543=DIRECTION ( 'NONE',  ( 0.000000000000000000, 0.000000000000000000, 1.000000000000000000 ) ) ;
#10544=CARTESIAN_POINT ( 'NONE',  ( -0.3013593406941685315, 0.3597456680659448791, 0.07637630773773090853 ) ) ;
#10564=CARTESIAN_POINT ( 'NONE',  ( -0.1669771619559717590, -0.4570419016572346282, 0.09284957166232934989 ) ) ;
#10566=CARTESIAN_POINT ( 'NONE',  ( -0.3412792617076849111, 0.05967164814832635888, 0.1377952755905512139 ) ) ;
#10567=AXIS2_PLACEMENT_3D ( 'NONE', #7032, #13511, #15527 ) ;
#10591=ORIENTED_EDGE ( 'NONE', *, *, #17152, .F. ) ;
#10593=AXIS2_PLACEMENT_3D ( 'NONE', #17982, #15631, #13086 ) ;
#10597=CARTESIAN_POINT ( 'NONE',  ( 0.2243804351485034487, 0.2666304421164708005, 0.1589462317787528611 ) ) ;
#10605=CARTESIAN_POINT ( 'NONE',  ( 6.557635703933409897E-17, 0.3771653543307084688, 0.07637549214372833795 ) ) ;
#10606=CARTESIAN_POINT ( 'NONE',  ( -0.3268939675028499914, -0.1881330340946393564, 0.07637795275590551769 ) ) ;
#10612=CARTESIAN_POINT ( 'NONE',  ( 0.1603262695921948977, -0.4410554214326551370, 0.07637549214372854611 ) ) ;
#10615=CIRCLE ( 'NONE', #24596, 0.4692913385826771866 ) ;
#10619=EDGE_CURVE ( 'NONE', #9720, #661, #11660, .T. ) ;
#10625=CARTESIAN_POINT ( 'NONE',  ( -0.3015429802558983741, -0.1746717017761129087, 0.1589462317904963562 ) ) ;
#10630=CARTESIAN_POINT ( 'NONE',  ( 0.3020979083622633565, 0.3591256245826334181, 0.07637795275590551769 ) ) ;
#10632=CARTESIAN_POINT ( 'NONE',  ( -0.3267210193396165585, -0.1884333032645074957, 0.1992150590373740204 ) ) ;
#10633=CARTESIAN_POINT ( 'NONE',  ( 0.000000000000000000, 0.000000000000000000, 0.07637795275590551769 ) ) ;
#10635=AXIS2_PLACEMENT_3D ( 'NONE', #20979, #6295, #27485 ) ;
#10646=CARTESIAN_POINT ( 'NONE',  ( 0.1715719712213541193, -0.4696414150092599882, 0.1259302777268271334 ) ) ;
#10654=CARTESIAN_POINT ( 'NONE',  ( -0.4620608682196457040, 0.08206165078054665496, 0.07637795275590551769 ) ) ;
#10659=CARTESIAN_POINT ( 'NONE',  ( -0.3019498226894488102, 0.3592501948414881796, 0.1992142434433716580 ) ) ;
#10670=ADVANCED_BREP_SHAPE_REPRESENTATION ( 'Deep Groove Ball Bearing 15x28x7', ( #21329, #11588 ), #2565 ) ;
#10685=ORIENTED_EDGE ( 'NONE', *, *, #22328, .F. ) ;
#10699=CARTESIAN_POINT ( 'NONE',  ( -0.1599629598573824862, -0.4411872753631803090, 0.07637795275590551769 ) ) ;
#10701=DIRECTION ( 'NONE',  ( 0.000000000000000000, 0.000000000000000000, 1.000000000000000000 ) ) ;
#10703=VERTEX_POINT ( 'NONE', #13783 ) ;
#10706=VERTEX_POINT ( 'NONE', #22403 ) ;
#10708=ORIENTED_EDGE ( 'NONE', *, *, #2574, .F. ) ;
#10743=DIRECTION ( 'NONE',  ( 0.000000000000000000, 0.000000000000000000, 1.000000000000000000 ) ) ;
#10753=CARTESIAN_POINT ( 'NONE',  ( -0.1189624676717062624, -0.3253923344978156829, 0.1276989850592374631 ) ) ;
#10761=DIRECTION ( 'NONE',  ( 0.000000000000000000, -1.000000000000000000, 0.000000000000000000 ) ) ;
#10774=CARTESIAN_POINT ( 'NONE',  ( -0.3263749705684267921, -0.1890319631540330891, 0.1992125984251968684 ) ) ;
#10801=CARTESIAN_POINT ( 'NONE',  ( -0.1608692170993913650, -0.4408576787418653775, 0.07637630773773071424 ) ) ;
#10814=AXIS2_PLACEMENT_3D ( 'NONE', #8204, #6096, #18378 ) ;
#10820=DIRECTION ( 'NONE',  ( 0.000000000000000000, 1.000000000000000000, 0.000000000000000000 ) ) ;
#10823=CARTESIAN_POINT ( 'NONE',  ( 0.0005847768872538051076, 0.4787829797961309919, 0.08349695147752299318 ) ) ;
#10825=ORIENTED_EDGE ( 'NONE', *, *, #24578, .F. ) ;
#10864=EDGE_CURVE ( 'NONE', #2522, #9569, #286, .T. ) ;
#10887=FACE_OUTER_BOUND ( 'NONE', #7619, .T. ) ;
#10891=DIRECTION ( 'NONE',  ( 0.000000000000000000, 0.000000000000000000, 1.000000000000000000 ) ) ;
#10892=CARTESIAN_POINT ( 'NONE',  ( 0.2236164729197613887, 0.2672714825449903908, 0.1589462317899844046 ) ) ;
#10894=CARTESIAN_POINT ( 'NONE',  ( -0.2428345617565149384, 0.2885915454824177218, 0.07637795275590551769 ) ) ;
#10900=VERTEX_POINT ( 'NONE', #17957 ) ;
#10904=VERTEX_POINT ( 'NONE', #24468 ) ;
#10910=CARTESIAN_POINT ( 'NONE',  ( 0.4622285577935897893, 0.08111201067594568659, 0.07637630773773071424 ) ) ;
#10916=ORIENTED_EDGE ( 'NONE', *, *, #26785, .F. ) ;
#10968=AXIS2_PLACEMENT_3D ( 'NONE', #12953, #19604, #8985 ) ;
#10970=ORIENTED_EDGE ( 'NONE', *, *, #608, .F. ) ;
#10976=ORIENTED_EDGE ( 'NONE', *, *, #25033, .F. ) ;
#10979=ORIENTED_EDGE ( 'NONE', *, *, #26249, .T. ) ;
#10983=ORIENTED_EDGE ( 'NONE', *, *, #24079, .T. ) ;
#10986=CARTESIAN_POINT ( 'NONE',  ( 0.3267210193396165585, -0.1884333032645078565, 0.1992150590373740204 ) ) ;
#11010=VERTEX_POINT ( 'NONE', #7682 ) ;
#11020=VERTEX_POINT ( 'NONE', #1324 ) ;
#11036=CARTESIAN_POINT ( 'NONE',  ( 0.2230788859036007821, 0.2650812153444456198, 0.1377952755905513527 ) ) ;
#11041=DIRECTION ( 'NONE',  ( 0.000000000000000000, 0.000000000000000000, 1.000000000000000000 ) ) ;
#11047=ORIENTED_EDGE ( 'NONE', *, *, #22758, .F. ) ;
#11051=CARTESIAN_POINT ( 'NONE',  ( 0.3411065095061436847, 0.06065137456822567580, 0.1276989850527261161 ) ) ;
#11053=CARTESIAN_POINT ( 'NONE',  ( -0.3100894960432669101, -0.1796141127297333773, 0.1805249803397054320 ) ) ;
#11057=DIRECTION ( 'NONE',  ( 0.000000000000000000, 1.000000000000000000, 0.000000000000000000 ) ) ;
#11058=CIRCLE ( 'NONE', #14212, 0.3771653543307086909 ) ;
#11060=DIRECTION ( 'NONE',  ( 0.000000000000000000, -1.000000000000000000, 0.000000000000000000 ) ) ;
#11079=CARTESIAN_POINT ( 'NONE',  ( 0.3268939675028499914, -0.1881330340946397728, 0.1992125984251968684 ) ) ;
#11101=EDGE_CURVE ( 'NONE', #6630, #20898, #13890, .T. ) ;
#11117=ORIENTED_EDGE ( 'NONE', *, *, #27640, .F. ) ;
#11134=EDGE_CURVE ( 'NONE', #21723, #19812, #586, .T. ) ;
#11140=ORIENTED_EDGE ( 'NONE', *, *, #1415, .F. ) ;
#11158=CARTESIAN_POINT ( 'NONE',  ( 0.1599629598573263645, -0.4411872753632007926, 0.1992125984251968684 ) ) ;
#11164=PLANE ( 'NONE',  #4657 ) ;
#11168=CARTESIAN_POINT ( 'NONE',  ( -5.645730259564185549E-17, 0.4692913385826772976, 0.07637549214372836570 ) ) ;
#11169=CARTESIAN_POINT ( 'NONE',  ( 0.3123213164505638240, 0.3731274149336368251, 0.1827409795199129161 ) ) ;
#11193=EDGE_CURVE ( 'NONE', #3390, #764, #6901, .T. ) ;
#11200=CARTESIAN_POINT ( 'NONE',  ( 0.3132247436403744478, 0.3723693495128845288, 0.1827409795189120778 ) ) ;
#11201=CARTESIAN_POINT ( 'NONE',  ( 0.1669771619565829646, -0.4570419016589117867, 0.09284957166463024547 ) ) ;
#11205=CARTESIAN_POINT ( 'NONE',  ( -0.4790936880893625349, 0.08507591033004376080, 0.09284957166262186590 ) ) ;
#11217=FACE_OUTER_BOUND ( 'NONE', #6930, .T. ) ;
#11237=DIRECTION ( 'NONE',  ( 0.000000000000000000, 0.000000000000000000, 1.000000000000000000 ) ) ;
#11253=ORIENTED_EDGE ( 'NONE', *, *, #1219, .T. ) ;
#11272=DIRECTION ( 'NONE',  ( 1.224646799147353207E-16, 1.000000000000000000, -0.000000000000000000 ) ) ;
#11283=VECTOR ( 'NONE', #12756, 39.37007874015748143 ) ;
#11287=EDGE_CURVE ( 'NONE', #12667, #27484, #15760, .T. ) ;
#11296=CARTESIAN_POINT ( 'NONE',  ( 0.3268939675028499914, -0.1881330340946397728, 0.07637795275590551769 ) ) ;
#11302=EDGE_CURVE ( 'NONE', #9249, #11890, #22245, .T. ) ;
#11304=EDGE_CURVE ( 'NONE', #17730, #8069, #24491, .T. ) ;
#11311=FACE_OUTER_BOUND ( 'NONE', #27357, .T. ) ;
#11316=DIRECTION ( 'NONE',  ( 0.000000000000000000, 0.000000000000000000, -1.000000000000000000 ) ) ;
#11317=EDGE_LOOP ( 'NONE', ( #6299, #22126, #12467, #18465 ) ) ;
#11329=TOROIDAL_SURFACE ( 'NONE', #1880, 0.4232283464566928832, 0.07677165354330708902 ) ;
#11330=FACE_OUTER_BOUND ( 'NONE', #1660, .T. ) ;
#11358=CARTESIAN_POINT ( 'NONE',  ( 0.2427018018350767803, 0.2887032559529629783, 0.07637630750536809898 ) ) ;
#11363=CIRCLE ( 'NONE', #19474, 0.07677362204724408334 ) ;
#11371=AXIS2_PLACEMENT_3D ( 'NONE', #4183, #14371, #16473 ) ;
#11379=DIRECTION ( 'NONE',  ( 0.000000000000000000, 0.000000000000000000, 1.000000000000000000 ) ) ;
#11384=DIRECTION ( 'NONE',  ( -0.6427876096865390299, 0.7660444431189783465, 0.000000000000000000 ) ) ;
#11388=ORIENTED_EDGE ( 'NONE', *, *, #16418, .T. ) ;
#11393=ORIENTED_EDGE ( 'NONE', *, *, #25719, .F. ) ;
#11403=AXIS2_PLACEMENT_3D ( 'NONE', #23848, #2349, #21991 ) ;
#11446=EDGE_CURVE ( 'NONE', #4298, #21302, #596, .T. ) ;
#11450=AXIS2_PLACEMENT_3D ( 'NONE', #4763, #11272, #19891 ) ;
#11477=CARTESIAN_POINT ( 'NONE',  ( 0.3715251363271980245, 0.06498290224717499786, 0.1992125984251968684 ) ) ;
#11488=AXIS2_PLACEMENT_3D ( 'NONE', #3609, #20153, #954 ) ;
#11503=DIRECTION ( 'NONE',  ( 0.000000000000000000, 1.000000000000000000, 0.000000000000000000 ) ) ;
#11512=ORIENTED_EDGE ( 'NONE', *, *, #17874, .F. ) ;
#11517=CIRCLE ( 'NONE', #19646, 0.3464566929133857665 ) ;
#11518=ORIENTED_EDGE ( 'NONE', *, *, #26098, .F. ) ;
#11523=ORIENTED_EDGE ( 'NONE', *, *, #211, .T. ) ;
#11527=ORIENTED_EDGE ( 'NONE', *, *, #16150, .T. ) ;
#11535=DIRECTION ( 'NONE',  ( 0.000000000000000000, 0.000000000000000000, 1.000000000000000000 ) ) ;
#11539=AXIS2_PLACEMENT_3D ( 'NONE', #21564, #25242, #23428 ) ;
#11546=AXIS2_PLACEMENT_3D ( 'NONE', #7496, #27418, #16395 ) ;
#11549=ORIENTED_EDGE ( 'NONE', *, *, #26249, .F. ) ;
#11554=( NAMED_UNIT ( * ) PLANE_ANGLE_UNIT ( ) SI_UNIT ( $, .RADIAN. ) ) ;
#11556=CARTESIAN_POINT ( 'NONE',  ( -0.4063220079890811354, -0.2348123150948578930, 0.07637549214372835182 ) ) ;
#11559=CARTESIAN_POINT ( 'NONE',  ( -0.3713448905834433322, 0.06600512665679449109, 0.07637795275590551769 ) ) ;
#11563=DIRECTION ( 'NONE',  ( 0.000000000000000000, 1.000000000000000000, 0.000000000000000000 ) ) ;
#11566=CIRCLE ( 'NONE', #2978, 0.07677362204724408334 ) ;
#11575=CARTESIAN_POINT ( 'NONE',  ( -0.1247869790649115962, -0.3443449117941754234, 0.08455817588007014107 ) ) ;
#11581=CARTESIAN_POINT ( 'NONE',  ( -0.3209354104561039089, 0.3834063931590963037, 0.1259302777217432279 ) ) ;
#11588=AXIS2_PLACEMENT_3D ( 'NONE', #5229, #3665, #7923 ) ;
#11589=ORIENTED_EDGE ( 'NONE', *, *, #3755, .T. ) ;
#11594=ORIENTED_EDGE ( 'NONE', *, *, #27605, .F. ) ;
#11600=B_SPLINE_CURVE_WITH_KNOTS ( 'NONE', 3,
 ( #26410, #451, #2408, #11168 ),
 .UNSPECIFIED., .F., .F.,
 ( 4, 4 ),
 ( 0.2376120521391529850, 0.2390783382518553157 ),
 .UNSPECIFIED. ) ;
#11609=CARTESIAN_POINT ( 'NONE',  ( -0.3715251363271980245, 0.06498290224717540031, 0.07637795275590551769 ) ) ;
#11613=CARTESIAN_POINT ( 'NONE',  ( 0.3714054139060134485, 0.06566393819133227450, 0.1992150590373740204 ) ) ;
#11623=ORIENTED_EDGE ( 'NONE', *, *, #3387, .T. ) ;
#11628=CARTESIAN_POINT ( 'NONE',  ( 0.4216927985374664400, -0.2427835582314127327, 0.1827409795180658381 ) ) ;
#11632=CARTESIAN_POINT ( 'NONE',  ( 0.000000000000000000, 0.000000000000000000, 0.01181102362204724393 ) ) ;
#11635=LINE ( 'NONE', #17585, #25772 ) ;
#11655=ORIENTED_EDGE ( 'NONE', *, *, #14788, .T. ) ;
#11660=LINE ( 'NONE', #21855, #4176 ) ;
#11665=CIRCLE ( 'NONE', #22502, 0.4692913385826771866 ) ;
#11672=DIRECTION ( 'NONE',  ( 0.000000000000000000, 0.000000000000000000, 1.000000000000000000 ) ) ;
#11685=SPHERICAL_SURFACE ( 'NONE', #15729, 0.07677362204724409722 ) ;
#11701=VERTEX_POINT ( 'NONE', #2894 ) ;
#11704=CARTESIAN_POINT ( 'NONE',  ( 0.4167985568850881561, 0.07349283109919291235, 0.1377952755905511861 ) ) ;
#11719=CARTESIAN_POINT ( 'NONE',  ( -0.1180276236025431524, -0.3257325899126714552, 0.1377952755905512139 ) ) ;
#11729=EDGE_CURVE ( 'NONE', #19036, #762, #3985, .T. ) ;
#11752=CARTESIAN_POINT ( 'NONE',  ( 0.1285103288269283661, -0.3545966721392122545, 0.07637795275590551769 ) ) ;
#11759=DIRECTION ( 'NONE',  ( 0.000000000000000000, 0.000000000000000000, 1.000000000000000000 ) ) ;
#11803=ORIENTED_EDGE ( 'NONE', *, *, #18215, .F. ) ;
#11834=EDGE_CURVE ( 'NONE', #496, #2802, #8677, .T. ) ;
#11840=DIRECTION ( 'NONE',  ( -0.9396926207859082059, 0.3420201433256689905, 0.000000000000000000 ) ) ;
#11852=DIRECTION ( 'NONE',  ( 0.000000000000000000, 1.000000000000000000, 0.000000000000000000 ) ) ;
#11882=EDGE_CURVE ( 'NONE', #19638, #27384, #26882, .T. ) ;
#11883=CIRCLE ( 'NONE', #4664, 0.3771653543307086909 ) ;
#11890=VERTEX_POINT ( 'NONE', #12228 ) ;
#11902=B_SPLINE_CURVE_WITH_KNOTS ( 'NONE', 3,
 ( #17255, #25872, #23900, #26144, #15431, #21911, #1994, #24023, #26274, #19508 ),
 .UNSPECIFIED., .F., .F.,
 ( 4, 2, 2, 2, 4 ),
 ( 0.000000000000000000, 0.2500000000000000000, 0.5000000000000000000, 0.7500000000000000000, 1.000000000000000000 ),
 .UNSPECIFIED. ) ;
#11908=ORIENTED_EDGE ( 'NONE', *, *, #25231, .F. ) ;
#11917=AXIS2_PLACEMENT_3D ( 'NONE', #4806, #584, #13701 ) ;
#11920=CARTESIAN_POINT ( 'NONE',  ( -0.1603262695921763847, -0.4410554214326614098, 0.1992150590373740204 ) ) ;
#11926=CARTESIAN_POINT ( 'NONE',  ( -0.3070866141732283561, 3.760726391082423050E-17, 0.2755905511811023723 ) ) ;
#11931=EDGE_CURVE ( 'NONE', #14590, #26957, #16261, .T. ) ;
#11960=CIRCLE ( 'NONE', #23247, 0.2952755905511810774 ) ;
#11991=TOROIDAL_SURFACE ( 'NONE', #6160, 0.4232283464566928832, 0.07677165354330708902 ) ;
#12007=CARTESIAN_POINT ( 'NONE',  ( 0.4067073728345488304, -0.2341441294389854655, 0.07637795275590551769 ) ) ;
#12011=CARTESIAN_POINT ( 'NONE',  ( 0.1601448837025137850, -0.4411213145380133982, 0.1992142434433712694 ) ) ;
#12027=AXIS2_PLACEMENT_3D ( 'NONE', #165, #22561, #17753 ) ;
#12029=CARTESIAN_POINT ( 'NONE',  ( 0.1187185187221477117, -0.3276343780125237637, 0.1589462317918231560 ) ) ;
#12031=DIRECTION ( 'NONE',  ( 0.000000000000000000, -1.000000000000000000, 0.000000000000000000 ) ) ;
#12034=LINE ( 'NONE', #3249, #27476 ) ;
#12038=DIRECTION ( 'NONE',  ( 1.000000000000000000, 0.000000000000000000, 0.000000000000000000 ) ) ;
#12055=CARTESIAN_POINT ( 'NONE',  ( 0.4067073728345788064, -0.2341441294389338956, 0.1992125984251968684 ) ) ;
#12059=TOROIDAL_SURFACE ( 'NONE', #27844, 0.4232283464566928832, 0.07677165354330708902 ) ;
#12063=SPHERICAL_SURFACE ( 'NONE', #27148, 0.07677362204724409722 ) ;
#12083=EDGE_CURVE ( 'NONE', #661, #8860, #5990, .T. ) ;
#12091=EDGE_LOOP ( 'NONE', ( #9686, #11623, #18619, #18563, #2793, #24065, #16988, #3432, #20037, #9041, #11, #25336, #8753 ) ) ;
#12115=ORIENTED_EDGE ( 'NONE', *, *, #17686, .F. ) ;
#12119=AXIS2_PLACEMENT_3D ( 'NONE', #21941, #17281, #2694 ) ;
#12123=CARTESIAN_POINT ( 'NONE',  ( 0.3015429802576074514, -0.1746717017771027003, 0.1166443193836266407 ) ) ;
#12126=VERTEX_POINT ( 'NONE', #10262 ) ;
#12130=DIRECTION ( 'NONE',  ( 0.000000000000000000, -1.000000000000000000, 0.000000000000000000 ) ) ;
#12132=AXIS2_PLACEMENT_3D ( 'NONE', #9306, #4667, #7348 ) ;
#12138=FACE_OUTER_BOUND ( 'NONE', #2532, .T. ) ;
#12156=DIRECTION ( 'NONE',  ( 0.000000000000000000, 0.000000000000000000, 1.000000000000000000 ) ) ;
#12166=CARTESIAN_POINT ( 'NONE',  ( -0.1288360683667815199, -0.3544784926413476200, 0.1992150590373740204 ) ) ;
#12169=CARTESIAN_POINT ( 'NONE',  ( -0.3174445073355823266, -0.1826860508809280137, 0.1910323753023780158 ) ) ;
#12170=CARTESIAN_POINT ( 'NONE',  ( -0.1257482708741702870, -0.3439950301908584196, 0.1910323753022282467 ) ) ;
#12172=DIRECTION ( 'NONE',  ( 0.000000000000000000, -1.000000000000000000, 0.000000000000000000 ) ) ;
#12174=CIRCLE ( 'NONE', #61, 0.5511811023622047445 ) ;
#12180=EDGE_CURVE ( 'NONE', #17997, #22192, #497, .T. ) ;
#12183=ORIENTED_EDGE ( 'NONE', *, *, #17152, .T. ) ;
#12188=EDGE_LOOP ( 'NONE', ( #5238, #20973, #20535, #9395 ) ) ;
#12191=CARTESIAN_POINT ( 'NONE',  ( 0.3174445073395564254, -0.1826860508832116869, 0.08455817587528674517 ) ) ;
#12192=CARTESIAN_POINT ( 'NONE',  ( 0.3013593406941988406, 0.3597456680659192330, 0.07637630773773071424 ) ) ;
#12206=EDGE_CURVE ( 'NONE', #23369, #6563, #394, .T. ) ;
#12220=VERTEX_POINT ( 'NONE', #2482 ) ;
#12228=CARTESIAN_POINT ( 'NONE',  ( 4.701028524955307180E-18, 0.4232283464566928832, 0.2145688976377952695 ) ) ;
#12231=ORIENTED_EDGE ( 'NONE', *, *, #27863, .F. ) ;
#12235=B_SPLINE_CURVE_WITH_KNOTS ( 'NONE', 3,
 ( #21255, #17022, #25629, #6668, #9043, #24164, #4799, #13416, #20061, #22739 ),
 .UNSPECIFIED., .F., .F.,
 ( 4, 2, 2, 2, 4 ),
 ( 0.000000000000000000, 0.2500000000000001665, 0.5000000000000003331, 0.7500000000000001110, 1.000000000000000000 ),
 .UNSPECIFIED. ) ;
#12261=ORIENTED_EDGE ( 'NONE', *, *, #25033, .T. ) ;
#12262=CIRCLE ( 'NONE', #26235, 0.5511811023622047445 ) ;
#12267=ORIENTED_EDGE ( 'NONE', *, *, #14581, .F. ) ;
#12272=CARTESIAN_POINT ( 'NONE',  ( -0.4622285577935968948, 0.08111201067590709246, 0.1992142434433716580 ) ) ;
#12274=EDGE_CURVE ( 'NONE', #240, #2204, #5928, .T. ) ;
#12290=FACE_OUTER_BOUND ( 'NONE', #2120, .T. ) ;
#12303=CARTESIAN_POINT ( 'NONE',  ( 0.1285103288269283661, -0.3545966721392122545, 0.1992125984251968684 ) ) ;
#12307=DIRECTION ( 'NONE',  ( -1.000000000000000000, 1.224646799147353454E-16, 0.000000000000000000 ) ) ;
#12309=CARTESIAN_POINT ( 'NONE',  ( 0.000000000000000000, 0.000000000000000000, 0.07637795275590551769 ) ) ;
#12317=CARTESIAN_POINT ( 'NONE',  ( -0.3263749705684267921, -0.1890319631540330891, 0.1992125984251968684 ) ) ;
#12319=CARTESIAN_POINT ( 'NONE',  ( 0.0005789221761214173069, 0.4692909815006417462, 0.07637795275590551769 ) ) ;
#12330=AXIS2_PLACEMENT_3D ( 'NONE', #24886, #18368, #12038 ) ;
#12334=CARTESIAN_POINT ( 'NONE',  ( -0.4167985568850881561, 0.07349283109919310664, 0.1377952755905511861 ) ) ;
#12337=CARTESIAN_POINT ( 'NONE',  ( -0.3607825703577880461, 0.06309631803640179670, 0.08455817587900750498 ) ) ;
#12341=DIRECTION ( 'NONE',  ( 0.000000000000000000, 0.000000000000000000, 1.000000000000000000 ) ) ;
#12348=VERTEX_POINT ( 'NONE', #7275 ) ;
#12349=AXIS2_PLACEMENT_3D ( 'NONE', #27079, #7727, #24941 ) ;
#12379=DIRECTION ( 'NONE',  ( 0.000000000000000000, 0.000000000000000000, 1.000000000000000000 ) ) ;
#12387=CIRCLE ( 'NONE', #8328, 0.4692913385826771866 ) ;
#12413=CARTESIAN_POINT ( 'NONE',  ( -0.3714952424334504455, 0.06515381386493838967, 0.1992142436757342316 ) ) ;
#12418=ORIENTED_EDGE ( 'NONE', *, *, #11729, .T. ) ;
#12421=CARTESIAN_POINT ( 'NONE',  ( 0.0005056364805146920096, 0.3583524373837443933, 0.09506557084337925734 ) ) ;
#12422=DIRECTION ( 'NONE',  ( 0.000000000000000000, 0.000000000000000000, -1.000000000000000000 ) ) ;
#12426=DIRECTION ( 'NONE',  ( 1.000000000000000000, 0.000000000000000000, 0.000000000000000000 ) ) ;
#12447=ADVANCED_FACE ( 'NONE', ( #9672 ), #11329, .F. ) ;
#12462=CARTESIAN_POINT ( 'NONE',  ( -0.3268939675028499914, -0.1881330340946393564, 0.1992125984251968684 ) ) ;
#12467=ORIENTED_EDGE ( 'NONE', *, *, #7794, .T. ) ;
#12521=DIRECTION ( 'NONE',  ( 0.000000000000000000, 0.000000000000000000, 1.000000000000000000 ) ) ;
#12526=DIRECTION ( 'NONE',  ( 0.000000000000000000, 0.000000000000000000, -1.000000000000000000 ) ) ;
#12532=CARTESIAN_POINT ( 'NONE',  ( 0.000000000000000000, 0.000000000000000000, 0.1377952755905511861 ) ) ;
#12539=CARTESIAN_POINT ( 'NONE',  ( -0.3015072509068622009, 0.3596217111731054850, 0.07637549214372835182 ) ) ;
#12551=ORIENTED_EDGE ( 'NONE', *, *, #211, .F. ) ;
#12560=CARTESIAN_POINT ( 'NONE',  ( -0.2421724791772047192, 0.2891474103999575052, 0.1992142436757342316 ) ) ;
#12575=VERTEX_POINT ( 'NONE', #21116 ) ;
#12584=ORIENTED_EDGE ( 'NONE', *, *, #13683, .T. ) ;
#12590=AXIS2_PLACEMENT_3D ( 'NONE', #9073, #8430, #24198 ) ;
#12596=VERTEX_POINT ( 'NONE', #1480 ) ;
#12603=CARTESIAN_POINT ( 'NONE',  ( 0.2427018018350767803, 0.2887032559529629783, 0.1992142436757342316 ) ) ;
#12605=EDGE_LOOP ( 'NONE', ( #5775, #5595, #18988, #19242, #2611, #19985 ) ) ;
#12626=TOROIDAL_SURFACE ( 'NONE', #457, 0.5393700787401575214, 0.01181102362204724393 ) ;
#12650=CARTESIAN_POINT ( 'NONE',  ( 0.4063220079890716430, -0.2348123150948751847, 0.1992150590373740204 ) ) ;
#12653=DIRECTION ( 'NONE',  ( 0.000000000000000000, 1.000000000000000000, 0.000000000000000000 ) ) ;
#12667=VERTEX_POINT ( 'NONE', #365 ) ;
#12675=ORIENTED_EDGE ( 'NONE', *, *, #5, .F. ) ;
#12680=EDGE_CURVE ( 'NONE', #27484, #15505, #19479, .T. ) ;
#12693=CARTESIAN_POINT ( 'NONE',  ( 0.3020416211906299941, -0.1738080303477508304, 0.1589462317999085772 ) ) ;
#12695=ADVANCED_FACE ( 'NONE', ( #237 ), #24067, .T. ) ;
#12718=CARTESIAN_POINT ( 'NONE',  ( 0.3268939675028499914, -0.1881330340946397728, 0.07637795275590551769 ) ) ;
#12728=CARTESIAN_POINT ( 'NONE',  ( 0.2299571666357553834, 0.2748389102014165974, 0.1805249803392612040 ) ) ;
#12730=ORIENTED_EDGE ( 'NONE', *, *, #20207, .F. ) ;
#12732=FACE_OUTER_BOUND ( 'NONE', #1801, .T. ) ;
#12748=DIRECTION ( 'NONE',  ( 0.000000000000000000, 0.000000000000000000, 1.000000000000000000 ) ) ;
#12755=CARTESIAN_POINT ( 'NONE',  ( 0.2223167940359795647, 0.2657206863494898097, 0.1276989850598370946 ) ) ;
#12756=DIRECTION ( 'NONE',  ( 0.000000000000000000, 0.000000000000000000, 1.000000000000000000 ) ) ;
#12783=EDGE_LOOP ( 'NONE', ( #23832, #25360, #3589, #15186 ) ) ;
#12836=CARTESIAN_POINT ( 'NONE',  ( 0.3105951325284482811, -0.1787383246579994367, 0.1805249803478745085 ) ) ;
#12859=CARTESIAN_POINT ( 'NONE',  ( 0.2230788859036006988, 0.2650812153444456754, 0.1478915661146933680 ) ) ;
#12862=CARTESIAN_POINT ( 'NONE',  ( 0.000000000000000000, 0.000000000000000000, 0.1377952755905511861 ) ) ;
#12870=DIRECTION ( 'NONE',  ( 1.000000000000000000, 0.000000000000000000, 0.000000000000000000 ) ) ;
#12893=CARTESIAN_POINT ( 'NONE',  ( -5.747161356628524594E-17, -0.4692913385826771866, 0.1992125984251968684 ) ) ;
#12895=CARTESIAN_POINT ( 'NONE',  ( 0.3665264996331779601, -0.2116141732283464416, 0.1377952755905511861 ) ) ;
#12902=ORIENTED_EDGE ( 'NONE', *, *, #23103, .T. ) ;
#12908=CARTESIAN_POINT ( 'NONE',  ( 0.1706130639248417957, -0.4670119966435259951, 0.1615162260935599503 ) ) ;
#12928=DIRECTION ( 'NONE',  ( 0.000000000000000000, 0.000000000000000000, 1.000000000000000000 ) ) ;
#12953=CARTESIAN_POINT ( 'NONE',  ( 0.000000000000000000, 0.000000000000000000, 0.2637795275590551491 ) ) ;
#12966=CIRCLE ( 'NONE', #788, 0.3771653543307086909 ) ;
#12968=CARTESIAN_POINT ( 'NONE',  ( 0.4895436826824360321, 0.08692528595286251603, 0.1140743250917607421 ) ) ;
#12991=ORIENTED_EDGE ( 'NONE', *, *, #15404, .T. ) ;
#12998=B_SPLINE_CURVE_WITH_KNOTS ( 'NONE', 3,
 ( #4654, #12859, #10597, #4116, #19363, #62 ),
 .UNSPECIFIED., .F., .F.,
 ( 4, 2, 4 ),
 ( 0.5000000000000000000, 0.7500000000000000000, 1.000000000000000000 ),
 .UNSPECIFIED. ) ;
#13022=ORIENTED_EDGE ( 'NONE', *, *, #23764, .F. ) ;
#13026=CARTESIAN_POINT ( 'NONE',  ( 0.4622619257814346572, 0.08092139668567618904, 0.07637795275590551769 ) ) ;
#13039=CARTESIAN_POINT ( 'NONE',  ( 0.000000000000000000, 0.000000000000000000, 0.1377952755905511861 ) ) ;
#13043=DIRECTION ( 'NONE',  ( 0.000000000000000000, -1.000000000000000000, 0.000000000000000000 ) ) ;
#13052=CARTESIAN_POINT ( 'NONE',  ( 0.1715719712208858272, -0.4696414150079809002, 0.1496602734630888831 ) ) ;
#13053=EDGE_CURVE ( 'NONE', #20876, #21486, #19943, .T. ) ;
#13085=ORIENTED_EDGE ( 'NONE', *, *, #20373, .F. ) ;
#13086=DIRECTION ( 'NONE',  ( 0.000000000000000000, 1.000000000000000000, 0.000000000000000000 ) ) ;
#13095=FACE_OUTER_BOUND ( 'NONE', #6604, .T. ) ;
#13100=EDGE_CURVE ( 'NONE', #2802, #14678, #575, .T. ) ;
#13105=CARTESIAN_POINT ( 'NONE',  ( -0.1706130639252569914, -0.4670119966446516502, 0.1140743250909571488 ) ) ;
#13106=AXIS2_PLACEMENT_3D ( 'NONE', #8010, #25229, #1640 ) ;
#13115=DIRECTION ( 'NONE',  ( 1.000000000000000000, 0.000000000000000000, 0.000000000000000000 ) ) ;
#13119=CARTESIAN_POINT ( 'NONE',  ( -5.645730259564185549E-17, 0.4692913385826772976, 0.07637549214372836570 ) ) ;
#13127=DIRECTION ( 'NONE',  ( 0.000000000000000000, 0.000000000000000000, 1.000000000000000000 ) ) ;
#13132=CARTESIAN_POINT ( 'NONE',  ( 0.000000000000000000, 0.000000000000000000, 0.1992125984251968684 ) ) ;
#13133=VERTEX_POINT ( 'NONE', #27788 ) ;
#13135=CARTESIAN_POINT ( 'NONE',  ( 0.2307318466679419144, 0.2741888764719463967, 0.09506557084205286001 ) ) ;
#13136=CARTESIAN_POINT ( 'NONE',  ( 0.000000000000000000, 0.000000000000000000, 0.1992125984251968684 ) ) ;
#13151=DIRECTION ( 'NONE',  ( 1.000000000000000000, 0.000000000000000000, 0.000000000000000000 ) ) ;
#13171=ADVANCED_FACE ( 'NONE', ( #17050 ), #20407, .F. ) ;
#13184=ORIENTED_EDGE ( 'NONE', *, *, #27786, .F. ) ;
#13192=AXIS2_PLACEMENT_3D ( 'NONE', #3136, #9493, #22937 ) ;
#13229=SPHERICAL_SURFACE ( 'NONE', #11403, 0.07677362204724409722 ) ;
#13272=ADVANCED_FACE ( 'NONE', ( #13482, #7134 ), #9102, .T. ) ;
#13273=CARTESIAN_POINT ( 'NONE',  ( -0.3665264996331779601, -0.2116141732283464416, 0.2145688976377952695 ) ) ;
#13274=CIRCLE ( 'NONE', #10567, 0.3771653543307086909 ) ;
#13280=CARTESIAN_POINT ( 'NONE',  ( 0.1704479274140477119, -0.4700505334956465164, 0.1496602734632995202 ) ) ;
#13305=CARTESIAN_POINT ( 'NONE',  ( 0.4621951630817676682, 0.08130208312401811244, 0.07637549214372854611 ) ) ;
#13308=CARTESIAN_POINT ( 'NONE',  ( -0.2997912780622380979, -0.1736589463928937815, 0.1377952755905510751 ) ) ;
#13310=AXIS2_PLACEMENT_3D ( 'NONE', #199, #1993, #8768 ) ;
#13312=CARTESIAN_POINT ( 'NONE',  ( 0.1180276236025431108, -0.3257325899126714552, 0.1377952755905513527 ) ) ;
#13339=CARTESIAN_POINT ( 'NONE',  ( -0.0005189969344232283309, 0.3771649972486724733, 0.1992125984251968684 ) ) ;
#13343=EDGE_CURVE ( 'NONE', #1560, #11010, #24133, .T. ) ;
#13376=ORIENTED_EDGE ( 'NONE', *, *, #3005, .F. ) ;
#13378=ADVANCED_FACE ( 'NONE', ( #18654 ), #14124, .F. ) ;
#13385=CARTESIAN_POINT ( 'NONE',  ( 0.000000000000000000, 0.000000000000000000, 0.1377952755905511861 ) ) ;
#13391=EDGE_CURVE ( 'NONE', #19933, #19454, #20075, .T. ) ;
#13395=EDGE_LOOP ( 'NONE', ( #10685, #8445, #13022, #4889, #11908, #18849 ) ) ;
#13400=CARTESIAN_POINT ( 'NONE',  ( 0.000000000000000000, 0.000000000000000000, 0.2755905511811023723 ) ) ;
#13406=ORIENTED_EDGE ( 'NONE', *, *, #6155, .F. ) ;
#13415=CARTESIAN_POINT ( 'NONE',  ( 6.557635703933409897E-17, 0.3771653543307084688, 0.07637549214372833795 ) ) ;
#13416=CARTESIAN_POINT ( 'NONE',  ( -0.3132247436399438478, 0.3723693495123709396, 0.1827409795197761921 ) ) ;
#13419=EDGE_CURVE ( 'NONE', #6563, #14294, #18133, .T. ) ;
#13438=ADVANCED_FACE ( 'NONE', ( #8089 ), #5069, .F. ) ;
#13441=CARTESIAN_POINT ( 'NONE',  ( -0.3665264996331779601, -0.2116141732283464416, 0.1377952755905511861 ) ) ;
#13463=B_SPLINE_CURVE_WITH_KNOTS ( 'NONE', 3,
 ( #25594, #23492, #12728, #10892, #21356, #19507 ),
 .UNSPECIFIED., .F., .F.,
 ( 4, 2, 4 ),
 ( 0.000000000000000000, 0.2500000000000000000, 0.5000000000000000000 ),
 .UNSPECIFIED. ) ;
#13482=FACE_BOUND ( 'NONE', #6780, .T. ) ;
#13491=CARTESIAN_POINT ( 'NONE',  ( 0.3607825703598260825, 0.06309631803675713746, 0.1910323753036465011 ) ) ;
#13511=DIRECTION ( 'NONE',  ( 0.000000000000000000, 0.000000000000000000, 1.000000000000000000 ) ) ;
#13520=CARTESIAN_POINT ( 'NONE',  ( 0.000000000000000000, 0.000000000000000000, 0.07637795275590551769 ) ) ;
#13531=CIRCLE ( 'NONE', #2693, 0.3771653543307086909 ) ;
#13550=DIRECTION ( 'NONE',  ( 0.1736481776669301369, -0.9848077530122081313, 0.000000000000000000 ) ) ;
#13559=CARTESIAN_POINT ( 'NONE',  ( -0.3123213164514010431, 0.3731274149346439639, 0.1827409795182249053 ) ) ;
#13562=CARTESIAN_POINT ( 'NONE',  ( -0.1288360683667815199, -0.3544784926413476200, 0.07637549214372835182 ) ) ;
#13589=DIRECTION ( 'NONE',  ( 0.000000000000000000, -1.000000000000000000, 0.000000000000000000 ) ) ;
#13602=B_SPLINE_CURVE_WITH_KNOTS ( 'NONE', 3,
 ( #11477, #613, #9481, #11613, #2708, #14951 ),
 .UNSPECIFIED., .F., .F.,
 ( 4, 2, 4 ),
 ( 0.6902184472752680433, 0.6915327610580710438, 0.6928470748408750435 ),
 .UNSPECIFIED. ) ;
#13608=ORIENTED_EDGE ( 'NONE', *, *, #2477, .T. ) ;
#13643=AXIS2_PLACEMENT_3D ( 'NONE', #7945, #16545, #2974 ) ;
#13649=VERTEX_POINT ( 'NONE', #23905 ) ;
#13669=EDGE_LOOP ( 'NONE', ( #9466, #21948, #4229, #3580, #9287, #16238 ) ) ;
#13677=AXIS2_PLACEMENT_3D ( 'NONE', #602, #7369, #4967 ) ;
#13683=EDGE_CURVE ( 'NONE', #14678, #661, #11600, .T. ) ;
#13701=DIRECTION ( 'NONE',  ( 0.000000000000000000, 1.000000000000000000, 0.000000000000000000 ) ) ;
#13706=EDGE_CURVE ( 'NONE', #25722, #9819, #21733, .T. ) ;
#13711=ORIENTED_EDGE ( 'NONE', *, *, #16246, .T. ) ;
#13734=CIRCLE ( 'NONE', #26829, 0.01181102362204724393 ) ;
#13741=ADVANCED_FACE ( 'NONE', ( #5073 ), #24059, .F. ) ;
#13783=CARTESIAN_POINT ( 'NONE',  ( 0.000000000000000000, 0.4692913385826771866, 0.2755905511811023723 ) ) ;
#13796=AXIS2_PLACEMENT_3D ( 'NONE', #22543, #9383, #26484 ) ;
#13817=ORIENTED_EDGE ( 'NONE', *, *, #8901, .T. ) ;
#13820=ORIENTED_EDGE ( 'NONE', *, *, #13419, .T. ) ;
#13822=ORIENTED_EDGE ( 'NONE', *, *, #22256, .F. ) ;
#13839=AXIS2_PLACEMENT_3D ( 'NONE', #26942, #16349, #20722 ) ;
#13850=CARTESIAN_POINT ( 'NONE',  ( -0.3100894960429780856, -0.1796141127295652340, 0.09506557084190404849 ) ) ;
#13851=ORIENTED_EDGE ( 'NONE', *, *, #12083, .F. ) ;
#13852=CIRCLE ( 'NONE', #20156, 0.4692913385826771866 ) ;
#13865=VERTEX_POINT ( 'NONE', #16252 ) ;
#13866=SPHERICAL_SURFACE ( 'NONE', #19820, 0.07677362204724409722 ) ;
#13877=CARTESIAN_POINT ( 'NONE',  ( 0.1180276236025431108, -0.3257325899126714552, 0.1377952755905513527 ) ) ;
#13878=CARTESIAN_POINT ( 'NONE',  ( 0.3020979083622633565, 0.3591256245826334181, 0.07637795275590551769 ) ) ;
#13890=LINE ( 'NONE', #5709, #27653 ) ;
#13896=CARTESIAN_POINT ( 'NONE',  ( 0.4308867145614553307, -0.2480839813576496411, 0.1140743250904989875 ) ) ;
#13929=VERTEX_POINT ( 'NONE', #10151 ) ;
#13944=CARTESIAN_POINT ( 'NONE',  ( -6.750021727583836750E-17, -0.5511811023622047445, 0.1377952755905511861 ) ) ;
#13948=DIRECTION ( 'NONE',  ( 1.000000000000000000, 0.000000000000000000, 0.000000000000000000 ) ) ;
#13989=CARTESIAN_POINT ( 'NONE',  ( 0.2720459371704843088, 0.3242117229735830830, 0.1377952755905511861 ) ) ;
#14008=DIRECTION ( 'NONE',  ( 0.000000000000000000, 0.000000000000000000, -1.000000000000000000 ) ) ;
#14009=VERTEX_POINT ( 'NONE', #14721 ) ;
#14011=( NAMED_UNIT ( * ) SI_UNIT ( $, .STERADIAN. ) SOLID_ANGLE_UNIT ( ) ) ;
#14016=VERTEX_POINT ( 'NONE', #27551 ) ;
#14046=SPHERICAL_SURFACE ( 'NONE', #1218, 0.07677362204724409722 ) ;
#14048=CARTESIAN_POINT ( 'NONE',  ( 0.3713752547280854133, 0.06583429795695137920, 0.07637630750536809898 ) ) ;
#14051=CARTESIAN_POINT ( 'NONE',  ( -0.2223167940359789541, 0.2657206863494903648, 0.1478915661187940878 ) ) ;
#14076=ORIENTED_EDGE ( 'NONE', *, *, #14941, .T. ) ;
#14080=B_SPLINE_CURVE_WITH_KNOTS ( 'NONE', 3,
 ( #19362, #21487, #25185, #5853, #12191, #12718 ),
 .UNSPECIFIED., .F., .F.,
 ( 4, 2, 4 ),
 ( 0.5000000000000000000, 0.7500000000000001110, 1.000000000000000000 ),
 .UNSPECIFIED. ) ;
#14081=CARTESIAN_POINT ( 'NONE',  ( 0.000000000000000000, 0.000000000000000000, 0.1377952755905511861 ) ) ;
#14083=DIRECTION ( 'NONE',  ( 0.000000000000000000, -1.000000000000000000, 0.000000000000000000 ) ) ;
#14102=VERTEX_POINT ( 'NONE', #2648 ) ;
#14121=CARTESIAN_POINT ( 'NONE',  ( 0.000000000000000000, 0.000000000000000000, 0.2637795275590551491 ) ) ;
#14124=TOROIDAL_SURFACE ( 'NONE', #13643, 0.4232283464566928832, 0.07677165354330708902 ) ;
#14131=DIRECTION ( 'NONE',  ( 1.000000000000000000, 0.000000000000000000, 0.000000000000000000 ) ) ;
#14136=CARTESIAN_POINT ( 'NONE',  ( -0.2236164729184980104, 0.2672714825434807095, 0.1166443193980749027 ) ) ;
#14141=ORIENTED_EDGE ( 'NONE', *, *, #22256, .T. ) ;
#14166=ADVANCED_FACE ( 'NONE', ( #4628 ), #5102, .F. ) ;
#14168=SPHERICAL_SURFACE ( 'NONE', #3327, 0.07677362204724409722 ) ;
#14170=CARTESIAN_POINT ( 'NONE',  ( -0.3020416211881005175, -0.1738080303462935516, 0.1589462317895919130 ) ) ;
#14174=EDGE_LOOP ( 'NONE', ( #23071, #25020, #25226, #15640 ) ) ;
#14212=AXIS2_PLACEMENT_3D ( 'NONE', #24223, #4861, #10820 ) ;
#14216=ORIENTED_EDGE ( 'NONE', *, *, #5033, .T. ) ;
#14249=FACE_BOUND ( 'NONE', #27052, .T. ) ;
#14266=AXIS2_PLACEMENT_3D ( 'NONE', #16215, #20297, #19154 ) ;
#14269=ORIENTED_EDGE ( 'NONE', *, *, #21194, .T. ) ;
#14271=CARTESIAN_POINT ( 'NONE',  ( 0.0004974201395668471654, 0.3464563358313494934, 0.1377952755905513249 ) ) ;
#14283=CARTESIAN_POINT ( 'NONE',  ( -0.2223167940359792594, 0.2657206863494902538, 0.1377952755905513249 ) ) ;
#14285=ORIENTED_EDGE ( 'NONE', *, *, #6699, .T. ) ;
#14294=VERTEX_POINT ( 'NONE', #20305 ) ;
#14297=CARTESIAN_POINT ( 'NONE',  ( -0.0005980912172654155416, 0.4999996422861965883, 0.1496602734623783681 ) ) ;
#14302=EDGE_CURVE ( 'NONE', #10388, #3132, #19571, .T. ) ;
#14305=DIRECTION ( 'NONE',  ( -0.9396926207859082059, 0.3420201433256691015, 0.000000000000000000 ) ) ;
#14308=ORIENTED_EDGE ( 'NONE', *, *, #3295, .F. ) ;
#14334=FACE_BOUND ( 'NONE', #25180, .T. ) ;
#14337=CARTESIAN_POINT ( 'NONE',  ( -0.3012109481301850633, 0.3598698725862389813, 0.07637795275590551769 ) ) ;
#14362=ORIENTED_EDGE ( 'NONE', *, *, #22572, .T. ) ;
#14371=DIRECTION ( 'NONE',  ( 0.9848077530122080203, -0.1736481776669309973, 0.000000000000000000 ) ) ;
#14378=VECTOR ( 'NONE', #19688, 39.37007874015748143 ) ;
#14389=DIRECTION ( 'NONE',  ( 1.000000000000000000, 0.000000000000000000, 0.000000000000000000 ) ) ;
#14391=FACE_OUTER_BOUND ( 'NONE', #79, .T. ) ;
#14399=ORIENTED_EDGE ( 'NONE', *, *, #22840, .T. ) ;
#14402=ORIENTED_EDGE ( 'NONE', *, *, #25712, .F. ) ;
#14422=CIRCLE ( 'NONE', #4486, 0.3771653543307086909 ) ;
#14423=UNCERTAINTY_MEASURE_WITH_UNIT (LENGTH_MEASURE( 1.000000000000000082E-05 ), #309, 'distance_accuracy_value', 'NONE') ;
#14427=MECHANICAL_DESIGN_GEOMETRIC_PRESENTATION_REPRESENTATION('',(#4915),#5845);
#14435=ADVANCED_FACE ( 'NONE', ( #3768 ), #23673, .T. ) ;
#14451=ORIENTED_EDGE ( 'NONE', *, *, #26649, .F. ) ;
#14461=DIRECTION ( 'NONE',  ( 0.000000000000000000, -1.000000000000000000, 0.000000000000000000 ) ) ;
#14480=CARTESIAN_POINT ( 'NONE',  ( 0.4067073728345488304, -0.2341441294389854655, 0.07637795275590551769 ) ) ;
#14491=ORIENTED_EDGE ( 'NONE', *, *, #14302, .F. ) ;
#14494=EDGE_CURVE ( 'NONE', #12596, #3390, #13602, .T. ) ;
#14496=AXIS2_PLACEMENT_3D ( 'NONE', #25929, #256, #6440 ) ;
#14511=CARTESIAN_POINT ( 'NONE',  ( 0.3020979083623086536, 0.3591256245825952265, 0.1992125984251968684 ) ) ;
#14529=CIRCLE ( 'NONE', #2310, 0.4692913385826771866 ) ;
#14535=DIRECTION ( 'NONE',  ( 0.000000000000000000, 0.000000000000000000, 1.000000000000000000 ) ) ;
#14537=DIRECTION ( 'NONE',  ( 0.000000000000000000, 0.000000000000000000, 1.000000000000000000 ) ) ;
#14554=CARTESIAN_POINT ( 'NONE',  ( -0.1694923354753281042, -0.4674199084430591400, 0.1140743250961406413 ) ) ;
#14559=B_SPLINE_CURVE_WITH_KNOTS ( 'NONE', 3,
 ( #15352, #25922, #21689, #13339 ),
 .UNSPECIFIED., .F., .F.,
 ( 4, 4 ),
 ( 0.6915327610580708217, 0.6928470748408740443 ),
 .UNSPECIFIED. ) ;
#14567=CARTESIAN_POINT ( 'NONE',  ( 0.4790936880894704486, 0.08507591033005897085, 0.09284957166276250340 ) ) ;
#14578=CARTESIAN_POINT ( 'NONE',  ( 0.1599629598573263645, -0.4411872753632007926, 0.1992125984251968684 ) ) ;
#14581=EDGE_CURVE ( 'NONE', #18025, #7189, #14992, .T. ) ;
#14590=VERTEX_POINT ( 'NONE', #22497 ) ;
#14594=CARTESIAN_POINT ( 'NONE',  ( 0.000000000000000000, 0.000000000000000000, 0.2637795275590551491 ) ) ;
#14623=DIRECTION ( 'NONE',  ( 0.000000000000000000, 0.000000000000000000, 1.000000000000000000 ) ) ;
#14632=CARTESIAN_POINT ( 'NONE',  ( 0.3018020646414338870, 0.3593743330771607125, 0.07637549214372835182 ) ) ;
#14636=DIRECTION ( 'NONE',  ( 1.000000000000000000, 0.000000000000000000, 0.000000000000000000 ) ) ;
#14661=CARTESIAN_POINT ( 'NONE',  ( 0.000000000000000000, 0.000000000000000000, 0.2755905511811023723 ) ) ;
#14676=EDGE_CURVE ( 'NONE', #14016, #6594, #27255, .T. ) ;
#14678=VERTEX_POINT ( 'NONE', #12319 ) ;
#14680=FACE_OUTER_BOUND ( 'NONE', #23535, .T. ) ;
#14683=ORIENTED_EDGE ( 'NONE', *, *, #18215, .T. ) ;
#14689=CIRCLE ( 'NONE', #8803, 0.07677362204724409722 ) ;
#14690=ORIENTED_EDGE ( 'NONE', *, *, #20264, .T. ) ;
#14691=ORIENTED_EDGE ( 'NONE', *, *, #22328, .T. ) ;
#14712=CARTESIAN_POINT ( 'NONE',  ( 0.4922996667773191226, 0.08741303158496288583, 0.1496602734591142292 ) ) ;
#14721=CARTESIAN_POINT ( 'NONE',  ( 0.4692913385826771866, 0.000000000000000000, 0.07637795275590551769 ) ) ;
#14726=CARTESIAN_POINT ( 'NONE',  ( -0.4622619257814346572, 0.08092139668567638333, 0.07637795275590551769 ) ) ;
#14740=CARTESIAN_POINT ( 'NONE',  ( -0.3528204557971049149, 0.06272520244115065147, 0.1805249803441617285 ) ) ;
#14741=DIRECTION ( 'NONE',  ( 0.000000000000000000, 1.000000000000000000, 0.000000000000000000 ) ) ;
#14742=ORIENTED_EDGE ( 'NONE', *, *, #11304, .F. ) ;
#14748=EDGE_CURVE ( 'NONE', #12348, #18025, #3796, .T. ) ;
#14757=CARTESIAN_POINT ( 'NONE',  ( 0.2425693455392318731, 0.2888145544500153594, 0.1992150590373740204 ) ) ;
#14762=VERTEX_POINT ( 'NONE', #2277 ) ;
#14768=CARTESIAN_POINT ( 'NONE',  ( -0.1187185187214592208, -0.3276343780106237280, 0.1589462317846821737 ) ) ;
#14776=CARTESIAN_POINT ( 'NONE',  ( -0.3412792617076848001, 0.05967164814832655317, 0.1276989850594592579 ) ) ;
#14780=DIRECTION ( 'NONE',  ( 0.000000000000000000, 1.000000000000000000, 0.000000000000000000 ) ) ;
#14786=CIRCLE ( 'NONE', #12027, 0.5393700787401575214 ) ;
#14788=EDGE_CURVE ( 'NONE', #13649, #2754, #22274, .T. ) ;
#14795=CARTESIAN_POINT ( 'NONE',  ( -0.1603262695921948977, -0.4410554214326551370, 0.07637549214372835182 ) ) ;
#14796=CIRCLE ( 'NONE', #23790, 0.3464566929133857665 ) ;
#14802=AXIS2_PLACEMENT_3D ( 'NONE', #1213, #11379, #22117 ) ;
#14821=DIRECTION ( 'NONE',  ( 0.000000000000000000, 1.000000000000000000, 0.000000000000000000 ) ) ;
#14826=VERTEX_POINT ( 'NONE', #25317 ) ;
#14836=ORIENTED_EDGE ( 'NONE', *, *, #21698, .F. ) ;
#14841=CARTESIAN_POINT ( 'NONE',  ( -0.1610509776512037416, -0.4407912692718771175, 0.07637795275590551769 ) ) ;
#14877=DIRECTION ( 'NONE',  ( 0.000000000000000000, -1.000000000000000000, 0.000000000000000000 ) ) ;
#14890=CARTESIAN_POINT ( 'NONE',  ( 0.1608692170993911430, -0.4408576787418653775, 0.07637630773773071424 ) ) ;
#14900=ADVANCED_FACE ( 'NONE', ( #11311 ), #22744, .T. ) ;
#14906=CARTESIAN_POINT ( 'NONE',  ( -0.2720459371704843088, 0.3242117229735834716, 0.2145688976377952695 ) ) ;
#14927=AXIS2_PLACEMENT_3D ( 'NONE', #1819, #5791, #10145 ) ;
#14930=CARTESIAN_POINT ( 'NONE',  ( 0.000000000000000000, 0.000000000000000000, 0.1377952755905511584 ) ) ;
#14941=EDGE_CURVE ( 'NONE', #3411, #25669, #18202, .T. ) ;
#14951=CARTESIAN_POINT ( 'NONE',  ( 0.3713448905834433322, 0.06600512665679410251, 0.1992125984251968684 ) ) ;
#14955=DIRECTION ( 'NONE',  ( 0.000000000000000000, -1.000000000000000000, 0.000000000000000000 ) ) ;
#14959=ORIENTED_EDGE ( 'NONE', *, *, #27786, .T. ) ;
#14968=ORIENTED_EDGE ( 'NONE', *, *, #8901, .F. ) ;
#14973=ORIENTED_EDGE ( 'NONE', *, *, #12274, .F. ) ;
#14992=B_SPLINE_CURVE_WITH_KNOTS ( 'NONE', 3,
 ( #24331, #2575, #11200, #9074, #17688, #20094, #7236, #26313, #15852, #13878 ),
 .UNSPECIFIED., .F., .F.,
 ( 4, 2, 2, 2, 4 ),
 ( 0.000000000000000000, 0.2500000000000001665, 0.5000000000000003331, 0.7500000000000001110, 1.000000000000000000 ),
 .UNSPECIFIED. ) ;
#14994=ORIENTED_EDGE ( 'NONE', *, *, #19595, .T. ) ;
#14996=( LENGTH_UNIT ( ) NAMED_UNIT ( * ) SI_UNIT ( $, .METRE. ) ) ;
#15000=CARTESIAN_POINT ( 'NONE',  ( 0.3528204557977369094, 0.06272520244126274236, 0.1805249803451361157 ) ) ;
#15011=ORIENTED_EDGE ( 'NONE', *, *, #20889, .T. ) ;
#15013=CARTESIAN_POINT ( 'NONE',  ( -5.747161356628524594E-17, -0.4692913385826771866, -3.278217716535432842E-17 ) ) ;
#15015=CIRCLE ( 'NONE', #11371, 0.07677362204724412498 ) ;
#15034=CARTESIAN_POINT ( 'NONE',  ( -0.2307318466671160750, 0.2741888764709654036, 0.1805249803371026529 ) ) ;
#15062=ORIENTED_EDGE ( 'NONE', *, *, #15544, .F. ) ;
#15063=CIRCLE ( 'NONE', #18149, 0.3070866141732283561 ) ;
#15081=EDGE_CURVE ( 'NONE', #16432, #9819, #9211, .T. ) ;
#15086=AXIS2_PLACEMENT_3D ( 'NONE', #3692, #3543, #12172 ) ;
#15100=ORIENTED_EDGE ( 'NONE', *, *, #5118, .T. ) ;
#15103=DIRECTION ( 'NONE',  ( 1.000000000000000000, 0.000000000000000000, 0.000000000000000000 ) ) ;
#15122=CARTESIAN_POINT ( 'NONE',  ( 0.3268939675028499914, -0.1881330340946397728, 0.1992125984251968684 ) ) ;
#15127=DIRECTION ( 'NONE',  ( 0.000000000000000000, 1.000000000000000000, 0.000000000000000000 ) ) ;
#15168=CARTESIAN_POINT ( 'NONE',  ( 0.000000000000000000, 0.000000000000000000, 0.1377952755905511861 ) ) ;
#15173=CARTESIAN_POINT ( 'NONE',  ( -0.2230788859036007821, 0.2650812153444458419, 0.1377952755905510474 ) ) ;
#15186=ORIENTED_EDGE ( 'NONE', *, *, #26961, .T. ) ;
#15190=CARTESIAN_POINT ( 'NONE',  ( -0.4895436826822647247, 0.08692528595283860460, 0.1615162260898340418 ) ) ;
#15198=ORIENTED_EDGE ( 'NONE', *, *, #11287, .T. ) ;
#15203=CARTESIAN_POINT ( 'NONE',  ( 0.2428345617565153547, 0.2885915454824177218, 0.07637795275590551769 ) ) ;
#15212=DIRECTION ( 'NONE',  ( 0.000000000000000000, 1.000000000000000000, 0.000000000000000000 ) ) ;
#15236=FACE_OUTER_BOUND ( 'NONE', #7178, .T. ) ;
#15243=ORIENTED_EDGE ( 'NONE', *, *, #20264, .F. ) ;
#15263=AXIS2_PLACEMENT_3D ( 'NONE', #23755, #21768, #4392 ) ;
#15291=FACE_OUTER_BOUND ( 'NONE', #20848, .T. ) ;
#15293=CARTESIAN_POINT ( 'NONE',  ( 0.000000000000000000, 0.000000000000000000, 0.1377952755905511861 ) ) ;
#15307=B_SPLINE_CURVE_WITH_KNOTS ( 'NONE', 3,
 ( #25723, #21901, #15000, #4387, #23890, #27848 ),
 .UNSPECIFIED., .F., .F.,
 ( 4, 2, 4 ),
 ( 0.000000000000000000, 0.2500000000000000000, 0.5000000000000000000 ),
 .UNSPECIFIED. ) ;
#15311=AXIS2_PLACEMENT_3D ( 'NONE', #9695, #9260, #2905 ) ;
#15320=ORIENTED_EDGE ( 'NONE', *, *, #18798, .T. ) ;
#15329=CARTESIAN_POINT ( 'NONE',  ( -0.5393700787401575214, 6.605378404849898113E-17, 0.2637795275590551491 ) ) ;
#15331=ORIENTED_EDGE ( 'NONE', *, *, #8643, .F. ) ;
#15335=AXIS2_PLACEMENT_3D ( 'NONE', #25933, #23555, #2696 ) ;
#15337=AXIS2_PLACEMENT_3D ( 'NONE', #17682, #13043, #4691 ) ;
#15344=ADVANCED_FACE ( 'NONE', ( #2516 ), #4371, .F. ) ;
#15352=CARTESIAN_POINT ( 'NONE',  ( 2.186367668367731174E-17, 0.3771653543307086909, 0.1992150590373740204 ) ) ;
#15355=CARTESIAN_POINT ( 'NONE',  ( 0.2425693455392318731, 0.2888145544500153594, 0.07637549214372835182 ) ) ;
#15363=DIRECTION ( 'NONE',  ( 1.000000000000000000, 0.000000000000000000, 0.000000000000000000 ) ) ;
#15375=CARTESIAN_POINT ( 'NONE',  ( -5.747161356628524594E-17, -0.4692913385826771866, 0.03818897637795275884 ) ) ;
#15379=AXIS2_PLACEMENT_3D ( 'NONE', #1420, #25152, #10035 ) ;
#15390=ORIENTED_EDGE ( 'NONE', *, *, #24463, .F. ) ;
#15391=ORIENTED_EDGE ( 'NONE', *, *, #24463, .T. ) ;
#15392=DIRECTION ( 'NONE',  ( 0.000000000000000000, 0.000000000000000000, -1.000000000000000000 ) ) ;
#15404=EDGE_CURVE ( 'NONE', #26363, #22611, #21868, .T. ) ;
#15415=ORIENTED_EDGE ( 'NONE', *, *, #14302, .T. ) ;
#15425=CARTESIAN_POINT ( 'NONE',  ( 0.1632039128460986976, -0.4501088385473325237, 0.08349695147770751225 ) ) ;
#15431=CARTESIAN_POINT ( 'NONE',  ( 0.4925073816792371884, 0.08623502184977957508, 0.1496602734459366590 ) ) ;
#15432=CARTESIAN_POINT ( 'NONE',  ( 0.000000000000000000, 0.000000000000000000, 0.1377952755905511584 ) ) ;
#15437=ORIENTED_EDGE ( 'NONE', *, *, #21075, .T. ) ;
#15450=VERTEX_POINT ( 'NONE', #21197 ) ;
#15451=CYLINDRICAL_SURFACE ( 'NONE', #5790, 0.4692913385826771866 ) ;
#15462=CIRCLE ( 'NONE', #3233, 0.4692913385826771866 ) ;
#15505=VERTEX_POINT ( 'NONE', #26221 ) ;
#15519=ORIENTED_EDGE ( 'NONE', *, *, #3755, .F. ) ;
#15520=ORIENTED_EDGE ( 'NONE', *, *, #3631, .T. ) ;
#15526=CARTESIAN_POINT ( 'NONE',  ( 0.000000000000000000, 0.000000000000000000, 0.1377952755905511861 ) ) ;
#15527=DIRECTION ( 'NONE',  ( 0.000000000000000000, 1.000000000000000000, 0.000000000000000000 ) ) ;
#15539=ORIENTED_EDGE ( 'NONE', *, *, #2085, .T. ) ;
#15544=EDGE_CURVE ( 'NONE', #16265, #6630, #11960, .T. ) ;
#15545=AXIS2_PLACEMENT_3D ( 'NONE', #1036, #25032, #26869 ) ;
#15559=SPHERICAL_SURFACE ( 'NONE', #19184, 0.07677362204724409722 ) ;
#15564=CARTESIAN_POINT ( 'NONE',  ( -0.4061284506583976994, -0.2351468520617070734, 0.1992125984251968684 ) ) ;
#15573=CIRCLE ( 'NONE', #10593, 0.4692913385826771866 ) ;
#15589=EDGE_CURVE ( 'NONE', #496, #10703, #1247, .T. ) ;
#15617=CARTESIAN_POINT ( 'NONE',  ( -0.1610509776512594748, -0.4407912692718567449, 0.1992125984251968684 ) ) ;
#15631=DIRECTION ( 'NONE',  ( 0.000000000000000000, 0.000000000000000000, 1.000000000000000000 ) ) ;
#15637=PRODUCT_DEFINITION_FORMATION_WITH_SPECIFIED_SOURCE ( 'ANY', '', #27402, .NOT_KNOWN. ) ;
#15640=ORIENTED_EDGE ( 'NONE', *, *, #8190, .F. ) ;
#15650=ORIENTED_EDGE ( 'NONE', *, *, #10391, .T. ) ;
#15675=TOROIDAL_SURFACE ( 'NONE', #367, 0.3070866141732283561, 0.01181102362204724393 ) ;
#15680=CARTESIAN_POINT ( 'NONE',  ( 0.1189624676717044721, -0.3253923344978163490, 0.1276989850526606129 ) ) ;
#15689=AXIS2_PLACEMENT_3D ( 'NONE', #4683, #19398, #2430 ) ;
#15692=CARTESIAN_POINT ( 'NONE',  ( 0.4063220079890811354, -0.2348123150948578930, 0.07637549214372854611 ) ) ;
#15702=EDGE_CURVE ( 'NONE', #27117, #4298, #2111, .T. ) ;
#15706=DIRECTION ( 'NONE',  ( 0.000000000000000000, -1.000000000000000000, 0.000000000000000000 ) ) ;
#15710=AXIS2_PLACEMENT_3D ( 'NONE', #16849, #16413, #25458 ) ;
#15716=ORIENTED_EDGE ( 'NONE', *, *, #16578, .F. ) ;
#15722=CARTESIAN_POINT ( 'NONE',  ( 0.0005189969344232283309, 0.3771649972486724733, 0.1992125984251968684 ) ) ;
#15729=AXIS2_PLACEMENT_3D ( 'NONE', #26507, #820, #9409 ) ;
#15743=EDGE_CURVE ( 'NONE', #3368, #4856, #24719, .T. ) ;
#15746=CARTESIAN_POINT ( 'NONE',  ( -0.4067073728345488304, -0.2341441294389850492, 0.07637795275590551769 ) ) ;
#15749=CIRCLE ( 'NONE', #2647, 0.3070866141732283561 ) ;
#15758=DIRECTION ( 'NONE',  ( -0.3420201433256691015, -0.9396926207859082059, 0.000000000000000000 ) ) ;
#15760=B_SPLINE_CURVE_WITH_KNOTS ( 'NONE', 3,
 ( #21787, #11051, #8921, #6818, #17548, #26162 ),
 .UNSPECIFIED., .F., .F.,
 ( 4, 2, 4 ),
 ( 0.5000000000000000000, 0.7500000000000000000, 1.000000000000000000 ),
 .UNSPECIFIED. ) ;
#15764=EDGE_LOOP ( 'NONE', ( #8984, #12267, #24586, #21167 ) ) ;
#15771=ORIENTED_EDGE ( 'NONE', *, *, #18379, .T. ) ;
#15782=FACE_OUTER_BOUND ( 'NONE', #16681, .T. ) ;
#15803=CARTESIAN_POINT ( 'NONE',  ( -0.4067073728345488304, -0.2341441294389850492, 0.07637795275590551769 ) ) ;
#15811=DIRECTION ( 'NONE',  ( 0.000000000000000000, 0.000000000000000000, 1.000000000000000000 ) ) ;
#15813=CARTESIAN_POINT ( 'NONE',  ( 0.1196556571320694373, -0.3272932875280350484, 0.1166443193822704893 ) ) ;
#15824=CIRCLE ( 'NONE', #14496, 0.3771653543307086909 ) ;
#15827=CARTESIAN_POINT ( 'NONE',  ( -0.1294857240059045234, -0.3542416573274181357, 0.07637795275590551769 ) ) ;
#15850=CARTESIAN_POINT ( 'NONE',  ( 0.0004986409324247901122, 0.3484797321232478429, 0.1589462317930195046 ) ) ;
#15852=CARTESIAN_POINT ( 'NONE',  ( 0.3082037322261920176, 0.3663931537946265582, 0.08349695147694113917 ) ) ;
#15890=ORIENTED_EDGE ( 'NONE', *, *, #26245, .T. ) ;
#15897=ORIENTED_EDGE ( 'NONE', *, *, #10391, .F. ) ;
#15903=ORIENTED_EDGE ( 'NONE', *, *, #7913, .F. ) ;
#15907=CARTESIAN_POINT ( 'NONE',  ( 0.1286734528930086607, -0.3545375539099149265, 0.1992142436757342316 ) ) ;
#15912=FACE_OUTER_BOUND ( 'NONE', #6105, .T. ) ;
#15927=AXIS2_PLACEMENT_3D ( 'NONE', #18337, #997, #14131 ) ;
#15947=ORIENTED_EDGE ( 'NONE', *, *, #6964, .T. ) ;
#15951=CARTESIAN_POINT ( 'NONE',  ( 0.1230388948667178323, -0.3365682031943129648, 0.09506557083416242171 ) ) ;
#15958=CARTESIAN_POINT ( 'NONE',  ( -0.4622619257814448712, 0.08092139668561793009, 0.1992125984251968684 ) ) ;
#15969=CARTESIAN_POINT ( 'NONE',  ( 0.1610509776512594748, -0.4407912692718567449, 0.1992125984251968684 ) ) ;
#15998=FACE_BOUND ( 'NONE', #1122, .T. ) ;
#16001=CARTESIAN_POINT ( 'NONE',  ( 0.1180276236025433051, -0.3257325899126712332, 0.1276989850574599683 ) ) ;
#16008=DIRECTION ( 'NONE',  ( 0.000000000000000000, 0.000000000000000000, 1.000000000000000000 ) ) ;
#16009=ORIENTED_EDGE ( 'NONE', *, *, #676, .F. ) ;
#16019=CARTESIAN_POINT ( 'NONE',  ( -0.4149306118461465465, -0.2388850582578584125, 0.08349695147705923914 ) ) ;
#16044=DIRECTION ( 'NONE',  ( 0.000000000000000000, 1.000000000000000000, 0.000000000000000000 ) ) ;
#16054=ORIENTED_EDGE ( 'NONE', *, *, #21603, .F. ) ;
#16087=B_SPLINE_CURVE_WITH_KNOTS ( 'NONE', 3,
 ( #21867, #6213, #1954, #19465, #25693, #4358, #13105, #10564, #21730, #14841 ),
 .UNSPECIFIED., .F., .F.,
 ( 4, 2, 2, 2, 4 ),
 ( 0.000000000000000000, 0.2499999999999998335, 0.4999999999999996669, 0.7499999999999997780, 1.000000000000000000 ),
 .UNSPECIFIED. ) ;
#16093=ORIENTED_EDGE ( 'NONE', *, *, #17507, .F. ) ;
#16106=CIRCLE ( 'NONE', #20619, 0.01181102362204724046 ) ;
#16107=FACE_OUTER_BOUND ( 'NONE', #7719, .T. ) ;
#16110=CARTESIAN_POINT ( 'NONE',  ( -0.3191377210039603174, 0.3812612458993721587, 0.1615162260891281343 ) ) ;
#16114=CARTESIAN_POINT ( 'NONE',  ( 2.186367668367731174E-17, 0.3771653543307086909, 0.1992150590373740204 ) ) ;
#16122=EDGE_CURVE ( 'NONE', #18410, #10904, #4748, .T. ) ;
#16128=CARTESIAN_POINT ( 'NONE',  ( -0.3411065095061437957, 0.06065137456822555090, 0.1377952755905512139 ) ) ;
#16139=EDGE_LOOP ( 'NONE', ( #9181, #14269 ) ) ;
#16143=CARTESIAN_POINT ( 'NONE',  ( -0.3713752547280854133, 0.06583429795695157349, 0.07637630750536809898 ) ) ;
#16146=VERTEX_POINT ( 'NONE', #2286 ) ;
#16150=EDGE_CURVE ( 'NONE', #339, #18410, #3116, .T. ) ;
#16155=ORIENTED_EDGE ( 'NONE', *, *, #17686, .T. ) ;
#16172=VERTEX_POINT ( 'NONE', #21934 ) ;
#16175=CARTESIAN_POINT ( 'NONE',  ( -5.747161356628524594E-17, -0.4692913385826771866, 0.2374015748031496065 ) ) ;
#16199=CIRCLE ( 'NONE', #27027, 0.4692913385826771866 ) ;
#16215=CARTESIAN_POINT ( 'NONE',  ( 0.1447526197146039584, -0.3977045540727763839, 0.1377952755905511861 ) ) ;
#16238=ORIENTED_EDGE ( 'NONE', *, *, #10013, .F. ) ;
#16244=DIRECTION ( 'NONE',  ( 0.000000000000000000, 0.000000000000000000, -1.000000000000000000 ) ) ;
#16245=DIRECTION ( 'NONE',  ( 0.000000000000000000, 0.000000000000000000, 1.000000000000000000 ) ) ;
#16246=EDGE_CURVE ( 'NONE', #26179, #20180, #4826, .T. ) ;
#16248=DIRECTION ( 'NONE',  ( 0.7660444431189775694, -0.6427876096865398070, 0.000000000000000000 ) ) ;
#16252=CARTESIAN_POINT ( 'NONE',  ( -0.4620608682196457040, 0.08206165078054665496, 0.07637795275590551769 ) ) ;
#16256=TOROIDAL_SURFACE ( 'NONE', #15689, 0.4232283464566928832, 0.07677165354330708902 ) ;
#16257=TOROIDAL_SURFACE ( 'NONE', #25268, 0.4232283464566928832, 0.07677165354330708902 ) ;
#16261=CIRCLE ( 'NONE', #9477, 0.07677362204724409722 ) ;
#16265=VERTEX_POINT ( 'NONE', #2426 ) ;
#16272=EDGE_CURVE ( 'NONE', #6594, #9793, #12174, .T. ) ;
#16278=DIRECTION ( 'NONE',  ( 0.000000000000000000, 0.000000000000000000, 1.000000000000000000 ) ) ;
#16281=VECTOR ( 'NONE', #137, 39.37007874015748143 ) ;
#16307=CARTESIAN_POINT ( 'NONE',  ( -0.2720459371704843088, 0.3242117229735834716, 0.1377952755905511861 ) ) ;
#16323=CARTESIAN_POINT ( 'NONE',  ( -0.4167985568850881561, 0.07349283109919312051, 0.06102165354330708891 ) ) ;
#16329=CARTESIAN_POINT ( 'NONE',  ( 0.3002886982018046491, -0.1727973894384566000, 0.1377952755905509363 ) ) ;
#16346=CARTESIAN_POINT ( 'NONE',  ( 0.000000000000000000, 0.2952755905511810774, 0.1377952755905511861 ) ) ;
#16349=DIRECTION ( 'NONE',  ( 0.000000000000000000, 0.000000000000000000, 1.000000000000000000 ) ) ;
#16368=CARTESIAN_POINT ( 'NONE',  ( -0.3263749705684267921, -0.1890319631540330891, 0.07637795275590551769 ) ) ;
#16393=EDGE_CURVE ( 'NONE', #26363, #8023, #7212, .T. ) ;
#16395=DIRECTION ( 'NONE',  ( -0.9396926207859082059, -0.3420201433256689905, 0.000000000000000000 ) ) ;
#16410=CARTESIAN_POINT ( 'NONE',  ( -0.1291602287245499914, -0.3543605079199910191, 0.1992150590373740204 ) ) ;
#16411=B_SPLINE_CURVE_WITH_KNOTS ( 'NONE', 3,
 ( #9962, #15907, #7568, #3030, #27073, #18564 ),
 .UNSPECIFIED., .F., .F.,
 ( 4, 2, 4 ),
 ( 0.6902184472752670441, 0.6915327610580710438, 0.6928470748408740443 ),
 .UNSPECIFIED. ) ;
#16413=DIRECTION ( 'NONE',  ( 0.000000000000000000, 0.000000000000000000, 1.000000000000000000 ) ) ;
#16414=AXIS2_PLACEMENT_3D ( 'NONE', #3652, #16810, #20903 ) ;
#16418=EDGE_CURVE ( 'NONE', #16265, #1951, #17154, .T. ) ;
#16432=VERTEX_POINT ( 'NONE', #8212 ) ;
#16438=CARTESIAN_POINT ( 'NONE',  ( 0.3714054139060134485, 0.06566393819133227450, 0.07637549214372835182 ) ) ;
#16452=ORIENTED_EDGE ( 'NONE', *, *, #10864, .T. ) ;
#16459=EDGE_CURVE ( 'NONE', #5280, #14016, #20759, .T. ) ;
#16464=ADVANCED_FACE ( 'NONE', ( #7931, #1290 ), #19075, .T. ) ;
#16473=DIRECTION ( 'NONE',  ( 0.1736481776669309418, 0.9848077530122079093, 0.000000000000000000 ) ) ;
#16482=CARTESIAN_POINT ( 'NONE',  ( 0.000000000000000000, 0.000000000000000000, 0.07637795275590551769 ) ) ;
#16493=ADVANCED_FACE ( 'NONE', ( #20921 ), #27547, .F. ) ;
#16534=CARTESIAN_POINT ( 'NONE',  ( -0.0005896702191535062526, 0.4865884552403880736, 0.1827409795202798448 ) ) ;
#16541=PRODUCT_DEFINITION ( 'UNKNOWN', '', #15637, #100 ) ;
#16544=EDGE_CURVE ( 'NONE', #11010, #240, #25781, .T. ) ;
#16545=DIRECTION ( 'NONE',  ( 0.000000000000000000, 0.000000000000000000, 1.000000000000000000 ) ) ;
#16566=EDGE_LOOP ( 'NONE', ( #13406, #20775, #1050, #11512, #387, #16009 ) ) ;
#16569=DIRECTION ( 'NONE',  ( 0.8660254037844387076, 0.4999999999999998890, -0.000000000000000000 ) ) ;
#16573=CARTESIAN_POINT ( 'NONE',  ( -0.3529960615001250801, 0.06172929298804197967, 0.09506557084278018099 ) ) ;
#16577=FACE_BOUND ( 'NONE', #26121, .T. ) ;
#16578=EDGE_CURVE ( 'NONE', #3390, #12667, #15307, .T. ) ;
#16586=B_SPLINE_CURVE_WITH_KNOTS ( 'NONE', 3,
 ( #10346, #5708, #16713, #14768, #23511, #25178 ),
 .UNSPECIFIED., .F., .F.,
 ( 4, 2, 4 ),
 ( 0.000000000000000000, 0.2500000000000000000, 0.5000000000000000000 ),
 .UNSPECIFIED. ) ;
#16619=CARTESIAN_POINT ( 'NONE',  ( 0.2997912780622382090, -0.1736589463928937538, 0.1377952755905513249 ) ) ;
#16623=CARTESIAN_POINT ( 'NONE',  ( 0.3073078020566822888, 0.3671449284701643889, 0.08349695147736714562 ) ) ;
#16628=FACE_OUTER_BOUND ( 'NONE', #9749, .T. ) ;
#16630=CARTESIAN_POINT ( 'NONE',  ( 0.000000000000000000, 0.000000000000000000, 0.1377952755905511861 ) ) ;
#16632=CARTESIAN_POINT ( 'NONE',  ( -0.3263749705684267921, -0.1890319631540330891, 0.07637795275590551769 ) ) ;
#16647=CARTESIAN_POINT ( 'NONE',  ( -0.0004974201395671521515, 0.3464563358313494934, 0.1377952755905512139 ) ) ;
#16665=CIRCLE ( 'NONE', #15337, 0.07677165354330708902 ) ;
#16681=EDGE_LOOP ( 'NONE', ( #17540, #12902 ) ) ;
#16682=CIRCLE ( 'NONE', #8114, 0.2952755905511810774 ) ;
#16692=CARTESIAN_POINT ( 'NONE',  ( -0.0005980912172688545225, 0.4999996422873391189, 0.1259302777261166184 ) ) ;
#16696=ORIENTED_EDGE ( 'NONE', *, *, #9036, .T. ) ;
#16713=CARTESIAN_POINT ( 'NONE',  ( -0.1220886091248651606, -0.3369140789097872513, 0.1805249803346592186 ) ) ;
#16717=ORIENTED_EDGE ( 'NONE', *, *, #3847, .T. ) ;
#16720=CARTESIAN_POINT ( 'NONE',  ( 0.000000000000000000, 0.000000000000000000, 0.1992125984251968684 ) ) ;
#16738=VERTEX_POINT ( 'NONE', #26527 ) ;
#16740=ORIENTED_EDGE ( 'NONE', *, *, #23246, .T. ) ;
#16746=EDGE_CURVE ( 'NONE', #24053, #26265, #10372, .T. ) ;
#16748=ORIENTED_EDGE ( 'NONE', *, *, #9458, .T. ) ;
#16749=ORIENTED_EDGE ( 'NONE', *, *, #5823, .F. ) ;
#16767=CARTESIAN_POINT ( 'NONE',  ( 0.3191377210032582123, 0.3812612458985252251, 0.1615162260922596571 ) ) ;
#16774=DIRECTION ( 'NONE',  ( 0.000000000000000000, 0.000000000000000000, -1.000000000000000000 ) ) ;
#16799=CARTESIAN_POINT ( 'NONE',  ( -0.2425693455392315123, 0.2888145544500153594, 0.1992150590373740204 ) ) ;
#16801=CARTESIAN_POINT ( 'NONE',  ( 0.4714076450718495126, 0.08371568475172405654, 0.08349695147687043184 ) ) ;
#16802=ORIENTED_EDGE ( 'NONE', *, *, #22850, .F. ) ;
#16810=DIRECTION ( 'NONE',  ( 0.000000000000000000, 1.000000000000000000, 0.000000000000000000 ) ) ;
#16818=EDGE_CURVE ( 'NONE', #19876, #27384, #8567, .T. ) ;
#16831=ORIENTED_EDGE ( 'NONE', *, *, #24508, .T. ) ;
#16834=ORIENTED_EDGE ( 'NONE', *, *, #11882, .F. ) ;
#16835=AXIS2_PLACEMENT_3D ( 'NONE', #17459, #15758, #21840 ) ;
#16836=CARTESIAN_POINT ( 'NONE',  ( 0.2952755905511810774, 0.000000000000000000, 0.01181102362204724393 ) ) ;
#16845=CARTESIAN_POINT ( 'NONE',  ( 0.000000000000000000, 0.000000000000000000, 0.1377952755905511861 ) ) ;
#16849=CARTESIAN_POINT ( 'NONE',  ( 0.000000000000000000, 0.000000000000000000, 0.2637795275590551491 ) ) ;
#16850=DIRECTION ( 'NONE',  ( 0.000000000000000000, 0.000000000000000000, -1.000000000000000000 ) ) ;
#16857=ORIENTED_EDGE ( 'NONE', *, *, #27605, .T. ) ;
#16869=DIRECTION ( 'NONE',  ( -0.9848077530122080203, 0.1736481776669311083, 0.000000000000000000 ) ) ;
#16875=ORIENTED_EDGE ( 'NONE', *, *, #15743, .F. ) ;
#16878=CARTESIAN_POINT ( 'NONE',  ( -0.3012109481301850633, 0.3598698725862389813, 0.1992125984251968684 ) ) ;
#16882=CARTESIAN_POINT ( 'NONE',  ( -0.4143458349595040002, -0.2398979215380011853, 0.08349695147757887903 ) ) ;
#16886=ORIENTED_EDGE ( 'NONE', *, *, #4386, .T. ) ;
#16895=CARTESIAN_POINT ( 'NONE',  ( 0.4067073728345788064, -0.2341441294389338956, 0.1992125984251968684 ) ) ;
#16912=DIRECTION ( 'NONE',  ( 1.000000000000000000, 0.000000000000000000, 0.000000000000000000 ) ) ;
#16919=ORIENTED_EDGE ( 'NONE', *, *, #14676, .T. ) ;
#16927=CARTESIAN_POINT ( 'NONE',  ( 0.000000000000000000, 0.000000000000000000, 0.1377952755905511584 ) ) ;
#16931=VERTEX_POINT ( 'NONE', #5428 ) ;
#16962=ADVANCED_FACE ( 'NONE', ( #18539 ), #12626, .T. ) ;
#16969=CARTESIAN_POINT ( 'NONE',  ( 0.000000000000000000, 0.000000000000000000, 0.01181102362204724393 ) ) ;
#16975=EDGE_CURVE ( 'NONE', #27484, #3132, #3445, .T. ) ;
#16988=ORIENTED_EDGE ( 'NONE', *, *, #25408, .F. ) ;
#17001=DIRECTION ( 'NONE',  ( 1.000000000000000000, 0.000000000000000000, 0.000000000000000000 ) ) ;
#17007=EDGE_LOOP ( 'NONE', ( #4992, #20561 ) ) ;
#17022=CARTESIAN_POINT ( 'NONE',  ( -0.3082037322265121504, 0.3663931537949983164, 0.08349695147730891442 ) ) ;
#17040=VERTEX_POINT ( 'NONE', #5855 ) ;
#17045=CARTESIAN_POINT ( 'NONE',  ( 0.5393700787401575214, 0.000000000000000000, -3.278217716535432842E-17 ) ) ;
#17050=FACE_OUTER_BOUND ( 'NONE', #2737, .T. ) ;
#17056=VERTEX_POINT ( 'NONE', #14906 ) ;
#17097=EDGE_LOOP ( 'NONE', ( #25066, #27875, #16740, #20600, #9704 ) ) ;
#17104=EDGE_CURVE ( 'NONE', #9793, #10277, #8391, .T. ) ;
#17106=ORIENTED_EDGE ( 'NONE', *, *, #18890, .T. ) ;
#17108=DIRECTION ( 'NONE',  ( 0.000000000000000000, 0.000000000000000000, 1.000000000000000000 ) ) ;
#17109=CIRCLE ( 'NONE', #2668, 0.3464566929133857665 ) ;
#17112=DIRECTION ( 'NONE',  ( 0.000000000000000000, 1.000000000000000000, 0.000000000000000000 ) ) ;
#17117=DIRECTION ( 'NONE',  ( 1.000000000000000000, 0.000000000000000000, 0.000000000000000000 ) ) ;
#17119=FACE_BOUND ( 'NONE', #8253, .T. ) ;
#17138=CARTESIAN_POINT ( 'NONE',  ( 0.000000000000000000, 0.000000000000000000, 0.2374015748031496065 ) ) ;
#17141=CARTESIAN_POINT ( 'NONE',  ( 0.1599629598573824862, -0.4411872753631803090, 0.07637795275590551769 ) ) ;
#17150=B_SPLINE_CURVE_WITH_KNOTS ( 'NONE', 3,
 ( #11752, #24455, #20232, #26720, #16001, #13877 ),
 .UNSPECIFIED., .F., .F.,
 ( 4, 2, 4 ),
 ( 0.000000000000000000, 0.2500000000000000000, 0.5000000000000000000 ),
 .UNSPECIFIED. ) ;
#17152=EDGE_CURVE ( 'NONE', #26179, #4298, #13531, .T. ) ;
#17154=CIRCLE ( 'NONE', #3663, 0.01181102362204724046 ) ;
#17155=CARTESIAN_POINT ( 'NONE',  ( 0.1610509776512594748, -0.4407912692718567449, 0.1992125984251968684 ) ) ;
#17161=ORIENTED_EDGE ( 'NONE', *, *, #11134, .F. ) ;
#17167=EDGE_CURVE ( 'NONE', #7189, #8124, #20330, .T. ) ;
#17199=VERTEX_POINT ( 'NONE', #14480 ) ;
#17200=CARTESIAN_POINT ( 'NONE',  ( -0.1632039128451868437, -0.4501088385448056006, 0.1920935997054097066 ) ) ;
#17219=ORIENTED_EDGE ( 'NONE', *, *, #18548, .F. ) ;
#17229=AXIS2_PLACEMENT_3D ( 'NONE', #26185, #8675, #25915 ) ;
#17234=ORIENTED_EDGE ( 'NONE', *, *, #16578, .T. ) ;
#17242=DIRECTION ( 'NONE',  ( 0.000000000000000000, 1.000000000000000000, 0.000000000000000000 ) ) ;
#17245=CARTESIAN_POINT ( 'NONE',  ( 0.2428345617565153547, 0.2885915454824177218, 0.07637795275590551769 ) ) ;
#17253=DIRECTION ( 'NONE',  ( -0.4999999999999995004, 0.8660254037844390407, 0.000000000000000000 ) ) ;
#17255=CARTESIAN_POINT ( 'NONE',  ( 0.4622619257814448712, 0.08092139668561752763, 0.1992125984251968684 ) ) ;
#17276=CARTESIAN_POINT ( 'NONE',  ( -0.3169330146481601496, -0.1835719822042344573, 0.1910323753027497184 ) ) ;
#17281=DIRECTION ( 'NONE',  ( 0.000000000000000000, 0.000000000000000000, 1.000000000000000000 ) ) ;
#17286=CARTESIAN_POINT ( 'NONE',  ( -0.4622619257814346572, 0.08092139668567638333, 0.07637795275590551769 ) ) ;
#17311=FACE_BOUND ( 'NONE', #24518, .T. ) ;
#17322=ADVANCED_FACE ( 'NONE', ( #8791 ), #16256, .F. ) ;
#17339=ORIENTED_EDGE ( 'NONE', *, *, #27470, .T. ) ;
#17363=EDGE_CURVE ( 'NONE', #23405, #11020, #2461, .T. ) ;
#17385=CARTESIAN_POINT ( 'NONE',  ( -0.3665264996331779601, -0.2116141732283464416, 0.06102165354330708891 ) ) ;
#17397=VERTEX_POINT ( 'NONE', #735 ) ;
#17401=EDGE_LOOP ( 'NONE', ( #5867, #15539, #15100, #22644 ) ) ;
#17415=ADVANCED_FACE ( 'NONE', ( #24731 ), #10249, .F. ) ;
#17431=DIRECTION ( 'NONE',  ( 0.000000000000000000, 0.000000000000000000, 1.000000000000000000 ) ) ;
#17436=CARTESIAN_POINT ( 'NONE',  ( 0.000000000000000000, 0.000000000000000000, 0.1992125984251968684 ) ) ;
#17442=DIRECTION ( 'NONE',  ( 0.3420201433256690460, -0.9396926207859084279, 0.000000000000000000 ) ) ;
#17458=VERTEX_POINT ( 'NONE', #16836 ) ;
#17459=CARTESIAN_POINT ( 'NONE',  ( -0.1447526197146041249, -0.3977045540727763839, 0.1377952755905511861 ) ) ;
#17461=ORIENTED_EDGE ( 'NONE', *, *, #5965, .T. ) ;
#17482=EDGE_CURVE ( 'NONE', #8860, #18722, #21642, .T. ) ;
#17497=TOROIDAL_SURFACE ( 'NONE', #22928, 0.4232283464566928832, 0.07677165354330708902 ) ;
#17507=EDGE_CURVE ( 'NONE', #27155, #8846, #4841, .T. ) ;
#17508=B_SPLINE_CURVE_WITH_KNOTS ( 'NONE', 3,
 ( #1394, #10014, #27544, #9873, #7768, #24985 ),
 .UNSPECIFIED., .F., .F.,
 ( 4, 2, 4 ),
 ( 0.7157687286427130147, 0.7172350147555660582, 0.7187013008684189908 ),
 .UNSPECIFIED. ) ;
#17518=ORIENTED_EDGE ( 'NONE', *, *, #16818, .F. ) ;
#17519=DIRECTION ( 'NONE',  ( 0.000000000000000000, 0.000000000000000000, 1.000000000000000000 ) ) ;
#17526=DIRECTION ( 'NONE',  ( 0.000000000000000000, 1.000000000000000000, 0.000000000000000000 ) ) ;
#17540=ORIENTED_EDGE ( 'NONE', *, *, #21194, .F. ) ;
#17541=CIRCLE ( 'NONE', #15335, 0.3464566929133857665 ) ;
#17542=ORIENTED_EDGE ( 'NONE', *, *, #23370, .F. ) ;
#17548=CARTESIAN_POINT ( 'NONE',  ( 0.3606049308168208234, 0.06410376196655420689, 0.08455817587496759768 ) ) ;
#17558=CARTESIAN_POINT ( 'NONE',  ( -0.3268939675028499914, -0.1881330340946393564, 0.1992125984251968684 ) ) ;
#17561=EDGE_CURVE ( 'NONE', #21486, #20876, #19317, .T. ) ;
#17585=CARTESIAN_POINT ( 'NONE',  ( 0.000000000000000000, 0.3771653543307086909, 0.03818897637795275884 ) ) ;
#17588=CARTESIAN_POINT ( 'NONE',  ( 0.000000000000000000, 0.000000000000000000, 0.1377952755905511584 ) ) ;
#17598=DIRECTION ( 'NONE',  ( 0.000000000000000000, 0.000000000000000000, 1.000000000000000000 ) ) ;
#17600=ADVANCED_FACE ( 'NONE', ( #22036 ), #26270, .T. ) ;
#17609=FACE_BOUND ( 'NONE', #6840, .T. ) ;
#17615=CARTESIAN_POINT ( 'NONE',  ( 0.3263749705684267921, -0.1890319631540330891, 0.1992125984251968684 ) ) ;
#17649=CARTESIAN_POINT ( 'NONE',  ( 0.1694923354742838562, -0.4674199084401557402, 0.1615162260937435257 ) ) ;
#17653=CIRCLE ( 'NONE', #9996, 0.4692913385826771866 ) ;
#17675=FACE_OUTER_BOUND ( 'NONE', #4423, .T. ) ;
#17679=FACE_OUTER_BOUND ( 'NONE', #5478, .T. ) ;
#17682=CARTESIAN_POINT ( 'NONE',  ( 0.4232283464566928832, 0.000000000000000000, 0.1377952755905511861 ) ) ;
#17686=EDGE_CURVE ( 'NONE', #22611, #12126, #24265, .T. ) ;
#17688=CARTESIAN_POINT ( 'NONE',  ( 0.3218517393630221934, 0.3826375019112421283, 0.1496602734594676132 ) ) ;
#17715=DIRECTION ( 'NONE',  ( 0.000000000000000000, 1.000000000000000000, 0.000000000000000000 ) ) ;
#17730=VERTEX_POINT ( 'NONE', #17903 ) ;
#17750=ORIENTED_EDGE ( 'NONE', *, *, #23162, .F. ) ;
#17753=DIRECTION ( 'NONE',  ( 0.000000000000000000, -1.000000000000000000, 0.000000000000000000 ) ) ;
#17756=ADVANCED_FACE ( 'NONE', ( #22171 ), #17497, .F. ) ;
#17761=FACE_OUTER_BOUND ( 'NONE', #16139, .T. ) ;
#17765=DIRECTION ( 'NONE',  ( 0.000000000000000000, 0.000000000000000000, 1.000000000000000000 ) ) ;
#17783=DIRECTION ( 'NONE',  ( 0.000000000000000000, 1.000000000000000000, 0.000000000000000000 ) ) ;
#17791=B_SPLINE_CURVE_WITH_KNOTS ( 'NONE', 3,
 ( #16647, #23152, #18888, #27387, #25257, #21021 ),
 .UNSPECIFIED., .F., .F.,
 ( 4, 2, 4 ),
 ( 0.5000000000000000000, 0.7500000000000000000, 1.000000000000000000 ),
 .UNSPECIFIED. ) ;
#17809=CIRCLE ( 'NONE', #13310, 0.07677362204724411110 ) ;
#17833=CYLINDRICAL_SURFACE ( 'NONE', #21923, 0.4692913385826771866 ) ;
#17869=CARTESIAN_POINT ( 'NONE',  ( 0.0001724821237275781839, 0.3771653543307086909, 0.1992150590373740204 ) ) ;
#17874=EDGE_CURVE ( 'NONE', #26931, #26179, #26667, .T. ) ;
#17876=LINE ( 'NONE', #13944, #404 ) ;
#17892=CARTESIAN_POINT ( 'NONE',  ( -0.4716107359529601584, 0.08256389912696107669, 0.1920935997046215038 ) ) ;
#17903=CARTESIAN_POINT ( 'NONE',  ( 0.1294857240059045234, -0.3542416573274181357, 0.07637795275590551769 ) ) ;
#17933=CARTESIAN_POINT ( 'NONE',  ( -0.3268939675028499914, -0.1881330340946393564, 0.07637795275590551769 ) ) ;
#17957=CARTESIAN_POINT ( 'NONE',  ( 0.1447526197146039584, -0.3977045540727763839, 0.06102165354330708891 ) ) ;
#17962=CARTESIAN_POINT ( 'NONE',  ( -0.4333114377119193783, -0.2494818589553494115, 0.1496602734600580575 ) ) ;
#17972=AXIS2_PLACEMENT_3D ( 'NONE', #6379, #10891, #21634 ) ;
#17979=EDGE_LOOP ( 'NONE', ( #11527, #4555, #6177, #23122 ) ) ;
#17981=ORIENTED_EDGE ( 'NONE', *, *, #14748, .F. ) ;
#17982=CARTESIAN_POINT ( 'NONE',  ( 0.000000000000000000, 0.000000000000000000, 0.07637795275590551769 ) ) ;
#17996=CARTESIAN_POINT ( 'NONE',  ( 2.186367668367731174E-17, 0.3771653543307086909, 0.1992150590373740204 ) ) ;
#17997=VERTEX_POINT ( 'NONE', #25696 ) ;
#18007=CIRCLE ( 'NONE', #14927, 0.4692913385826771866 ) ;
#18020=CARTESIAN_POINT ( 'NONE',  ( -0.3070866141732283561, 3.760726391082423050E-17, -1.639108858267716421E-17 ) ) ;
#18022=CARTESIAN_POINT ( 'NONE',  ( -0.2952755905511810774, 3.688404729715453115E-17, 0.2637795275590551491 ) ) ;
#18025=VERTEX_POINT ( 'NONE', #21595 ) ;
#18040=CARTESIAN_POINT ( 'NONE',  ( -0.0004974201395671521515, 0.3464563358313494934, 0.1377952755905512139 ) ) ;
#18046=CIRCLE ( 'NONE', #5924, 0.07677165354330708902 ) ;
#18050=CARTESIAN_POINT ( 'NONE',  ( 0.000000000000000000, 0.000000000000000000, 0.1377952755905511861 ) ) ;
#18063=CARTESIAN_POINT ( 'NONE',  ( -0.3002886982018051487, -0.1727973894384557951, 0.1276989850589877462 ) ) ;
#18073=CARTESIAN_POINT ( 'NONE',  ( -0.1286734528930088550, -0.3545375539099149265, 0.1992142436757342316 ) ) ;
#18076=EDGE_CURVE ( 'NONE', #9249, #11890, #19339, .T. ) ;
#18086=EDGE_LOOP ( 'NONE', ( #4261, #21512 ) ) ;
#18094=CARTESIAN_POINT ( 'NONE',  ( 0.4333114377119646754, -0.2494818589553824129, 0.1259302777214051094 ) ) ;
#18099=B_SPLINE_CURVE_WITH_KNOTS ( 'NONE', 3,
 ( #2680, #3090, #13562, #582, #20066, #15827 ),
 .UNSPECIFIED., .F., .F.,
 ( 4, 2, 4 ),
 ( 0.2291966065698869959, 0.2305109203526899964, 0.2318252341354939960 ),
 .UNSPECIFIED. ) ;
#18100=DIRECTION ( 'NONE',  ( 0.000000000000000000, 0.000000000000000000, 1.000000000000000000 ) ) ;
#18117=DIRECTION ( 'NONE',  ( 0.000000000000000000, 0.000000000000000000, 1.000000000000000000 ) ) ;
#18120=CARTESIAN_POINT ( 'NONE',  ( 0.3715251363271980245, 0.06498290224717499786, 0.1992125984251968684 ) ) ;
#18133=CIRCLE ( 'NONE', #19959, 0.4692913385826771866 ) ;
#18138=ORIENTED_EDGE ( 'NONE', *, *, #1415, .T. ) ;
#18139=CARTESIAN_POINT ( 'NONE',  ( -0.2428345617565149384, 0.2885915454824177218, 0.07637795275590551769 ) ) ;
#18141=EDGE_CURVE ( 'NONE', #14016, #5387, #17876, .T. ) ;
#18148=ADVANCED_FACE ( 'NONE', ( #3038 ), #3054, .F. ) ;
#18149=AXIS2_PLACEMENT_3D ( 'NONE', #25158, #3979, #12031 ) ;
#18202=CIRCLE ( 'NONE', #11917, 0.3771653543307086909 ) ;
#18215=EDGE_CURVE ( 'NONE', #16146, #12126, #25373, .T. ) ;
#18216=CARTESIAN_POINT ( 'NONE',  ( -0.3020416211876971735, -0.1738080303460615705, 0.1166443193931544220 ) ) ;
#18222=CIRCLE ( 'NONE', #8774, 0.4692913385826771866 ) ;
#18224=ORIENTED_EDGE ( 'NONE', *, *, #25231, .T. ) ;
#18229=FACE_OUTER_BOUND ( 'NONE', #17097, .T. ) ;
#18248=DIRECTION ( 'NONE',  ( 0.000000000000000000, 0.000000000000000000, -1.000000000000000000 ) ) ;
#18253=DIRECTION ( 'NONE',  ( 0.000000000000000000, 0.000000000000000000, 1.000000000000000000 ) ) ;
#18262=EDGE_LOOP ( 'NONE', ( #21858, #25085, #26918, #10708, #25496, #13851 ) ) ;
#18267=ADVANCED_FACE ( 'NONE', ( #25232 ), #421, .F. ) ;
#18308=DIRECTION ( 'NONE',  ( 0.9396926207859082059, -0.3420201433256690460, 0.000000000000000000 ) ) ;
#18315=ORIENTED_EDGE ( 'NONE', *, *, #27546, .T. ) ;
#18318=FACE_OUTER_BOUND ( 'NONE', #8997, .T. ) ;
#18320=CARTESIAN_POINT ( 'NONE',  ( 0.2997912780622382090, -0.1736589463928937538, 0.1377952755905513249 ) ) ;
#18322=ORIENTED_EDGE ( 'NONE', *, *, #6699, .F. ) ;
#18325=ORIENTED_EDGE ( 'NONE', *, *, #6361, .F. ) ;
#18331=CARTESIAN_POINT ( 'NONE',  ( 0.4167985568850881561, 0.07349283109919289847, 0.2145688976377952695 ) ) ;
#18334=CARTESIAN_POINT ( 'NONE',  ( -0.1180276236025431524, -0.3257325899126714552, 0.1377952755905512139 ) ) ;
#18337=CARTESIAN_POINT ( 'NONE',  ( 0.000000000000000000, 0.000000000000000000, 0.1377952755905511861 ) ) ;
#18338=CARTESIAN_POINT ( 'NONE',  ( -0.3073078020560655044, 0.3671449284694313087, 0.08349695147664858152 ) ) ;
#18341=CARTESIAN_POINT ( 'NONE',  ( -0.2350342994816159436, 0.2808987121518214392, 0.08455817588142111596 ) ) ;
#18368=DIRECTION ( 'NONE',  ( 0.000000000000000000, 0.000000000000000000, 1.000000000000000000 ) ) ;
#18373=ORIENTED_EDGE ( 'NONE', *, *, #7491, .T. ) ;
#18374=B_SPLINE_CURVE_WITH_KNOTS ( 'NONE', 3,
 ( #24691, #15680, #15813, #15951, #9161, #20183 ),
 .UNSPECIFIED., .F., .F.,
 ( 4, 2, 4 ),
 ( 0.5000000000000000000, 0.7500000000000000000, 1.000000000000000000 ),
 .UNSPECIFIED. ) ;
#18378=DIRECTION ( 'NONE',  ( 0.000000000000000000, 0.000000000000000000, -1.000000000000000000 ) ) ;
#18379=EDGE_CURVE ( 'NONE', #12220, #9015, #17541, .T. ) ;
#18393=DIRECTION ( 'NONE',  ( -0.6427876096865393629, 0.7660444431189780135, 0.000000000000000000 ) ) ;
#18395=CIRCLE ( 'NONE', #8935, 0.5393700787401575214 ) ;
#18400=CARTESIAN_POINT ( 'NONE',  ( 0.000000000000000000, 0.000000000000000000, 0.1377952755905511584 ) ) ;
#18403=B_SPLINE_CURVE_WITH_KNOTS ( 'NONE', 3,
 ( #22607, #5228, #8167, #13850, #10263, #3227 ),
 .UNSPECIFIED., .F., .F.,
 ( 4, 2, 4 ),
 ( 0.5000000000000000000, 0.7500000000000002220, 1.000000000000000000 ),
 .UNSPECIFIED. ) ;
#18410=VERTEX_POINT ( 'NONE', #25519 ) ;
#18412=ADVANCED_FACE ( 'NONE', ( #11330 ), #19946, .T. ) ;
#18424=ORIENTED_EDGE ( 'NONE', *, *, #16393, .F. ) ;
#18430=SPHERICAL_SURFACE ( 'NONE', #12349, 0.07677362204724409722 ) ;
#18439=FACE_OUTER_BOUND ( 'NONE', #11317, .T. ) ;
#18465=ORIENTED_EDGE ( 'NONE', *, *, #18731, .T. ) ;
#18467=ORIENTED_EDGE ( 'NONE', *, *, #22413, .F. ) ;
#18492=EDGE_CURVE ( 'NONE', #5345, #1951, #15749, .T. ) ;
#18493=ORIENTED_EDGE ( 'NONE', *, *, #676, .T. ) ;
#18496=ORIENTED_EDGE ( 'NONE', *, *, #6857, .F. ) ;
#18497=CARTESIAN_POINT ( 'NONE',  ( -0.3070866141732283561, 3.760726391082423050E-17, 0.01181102362204724393 ) ) ;
#18511=EDGE_CURVE ( 'NONE', #3709, #17997, #20580, .T. ) ;
#18521=ORIENTED_EDGE ( 'NONE', *, *, #17482, .T. ) ;
#18539=FACE_OUTER_BOUND ( 'NONE', #7154, .T. ) ;
#18548=EDGE_CURVE ( 'NONE', #26883, #10706, #22270, .T. ) ;
#18553=ORIENTED_EDGE ( 'NONE', *, *, #13053, .T. ) ;
#18563=ORIENTED_EDGE ( 'NONE', *, *, #608, .T. ) ;
#18564=CARTESIAN_POINT ( 'NONE',  ( 0.1294857240059045234, -0.3542416573274181357, 0.1992125984251968684 ) ) ;
#18566=EDGE_LOOP ( 'NONE', ( #5711, #16748, #19162, #135, #20108, #8705, #10158, #17981, #10162, #26934, #4409, #1352, #17518, #26424 ) ) ;
#18591=DIRECTION ( 'NONE',  ( -0.3420201433256691570, -0.9396926207859082059, 0.000000000000000000 ) ) ;
#18598=CARTESIAN_POINT ( 'NONE',  ( 0.000000000000000000, 0.000000000000000000, 0.1377952755905511584 ) ) ;
#18614=VECTOR ( 'NONE', #5437, 39.37007874015748143 ) ;
#18619=ORIENTED_EDGE ( 'NONE', *, *, #169, .F. ) ;
#18642=ORIENTED_EDGE ( 'NONE', *, *, #11193, .T. ) ;
#18645=DIRECTION ( 'NONE',  ( 1.000000000000000000, 0.000000000000000000, 0.000000000000000000 ) ) ;
#18654=FACE_OUTER_BOUND ( 'NONE', #14174, .T. ) ;
#18657=CARTESIAN_POINT ( 'NONE',  ( 0.2428345617565153547, 0.2885915454824177218, 0.1992125984251968684 ) ) ;
#18659=CARTESIAN_POINT ( 'NONE',  ( -4.618943439303797186E-17, -0.3771653543307086909, 0.1992125984251968684 ) ) ;
#18712=AXIS2_PLACEMENT_3D ( 'NONE', #19444, #10543, #14821 ) ;
#18720=B_SPLINE_CURVE_WITH_KNOTS ( 'NONE', 3,
 ( #22922, #25028, #14170, #5692, #12169, #12462 ),
 .UNSPECIFIED., .F., .F.,
 ( 4, 2, 4 ),
 ( 0.5000000000000000000, 0.7500000000000001110, 1.000000000000000000 ),
 .UNSPECIFIED. ) ;
#18722=VERTEX_POINT ( 'NONE', #3345 ) ;
#18731=EDGE_CURVE ( 'NONE', #7534, #9015, #5416, .T. ) ;
#18739=DIRECTION ( 'NONE',  ( 0.000000000000000000, 0.000000000000000000, 1.000000000000000000 ) ) ;
#18754=ORIENTED_EDGE ( 'NONE', *, *, #17507, .T. ) ;
#18763=DIRECTION ( 'NONE',  ( -0.8660254037844390407, -0.4999999999999994449, 0.000000000000000000 ) ) ;
#18770=FACE_BOUND ( 'NONE', #3662, .T. ) ;
#18781=DIRECTION ( 'NONE',  ( -1.000000000000000000, 0.000000000000000000, 0.000000000000000000 ) ) ;
#18786=DIRECTION ( 'NONE',  ( 1.000000000000000000, 0.000000000000000000, 0.000000000000000000 ) ) ;
#18795=ORIENTED_EDGE ( 'NONE', *, *, #7913, .T. ) ;
#18798=EDGE_CURVE ( 'NONE', #762, #22736, #14559, .T. ) ;
#18817=ORIENTED_EDGE ( 'NONE', *, *, #12680, .T. ) ;
#18842=ORIENTED_EDGE ( 'NONE', *, *, #5, .T. ) ;
#18849=ORIENTED_EDGE ( 'NONE', *, *, #18731, .F. ) ;
#18860=AXIS2_PLACEMENT_3D ( 'NONE', #15526, #11535, #812 ) ;
#18871=EDGE_CURVE ( 'NONE', #3411, #25722, #1361, .T. ) ;
#18872=ORIENTED_EDGE ( 'NONE', *, *, #5090, .F. ) ;
#18875=CARTESIAN_POINT ( 'NONE',  ( 0.3412792617076850221, 0.05967164814832588010, 0.1377952755905512139 ) ) ;
#18888=CARTESIAN_POINT ( 'NONE',  ( -0.0004986409324230409688, 0.3484797321218884303, 0.1166443193928871913 ) ) ;
#18890=EDGE_CURVE ( 'NONE', #8023, #25040, #16106, .T. ) ;
#18900=CARTESIAN_POINT ( 'NONE',  ( -0.2420394123212937232, 0.2892587550802429575, 0.1992125984251968684 ) ) ;
#18903=B_SPLINE_CURVE_WITH_KNOTS ( 'NONE', 3,
 ( #5964, #25155, #12029, #9761, #22911, #12303 ),
 .UNSPECIFIED., .F., .F.,
 ( 4, 2, 4 ),
 ( 0.5000000000000000000, 0.7500000000000000000, 1.000000000000000000 ),
 .UNSPECIFIED. ) ;
#18943=ADVANCED_FACE ( 'NONE', ( #4399 ), #2110, .F. ) ;
#18948=SPHERICAL_SURFACE ( 'NONE', #23282, 0.07677362204724409722 ) ;
#18961=DIRECTION ( 'NONE',  ( 0.000000000000000000, 1.000000000000000000, 0.000000000000000000 ) ) ;
#18962=ADVANCED_FACE ( 'NONE', ( #8496 ), #24203, .F. ) ;
#18963=EDGE_CURVE ( 'NONE', #2754, #13649, #14786, .T. ) ;
#18968=CARTESIAN_POINT ( 'NONE',  ( 0.2299571666351564181, 0.2748389102007000040, 0.09506557084325908957 ) ) ;
#18978=ADVANCED_FACE ( 'NONE', ( #18439 ), #19245, .F. ) ;
#18979=ORIENTED_EDGE ( 'NONE', *, *, #10619, .T. ) ;
#18984=CARTESIAN_POINT ( 'NONE',  ( 0.3012109481301854519, 0.3598698725862389813, 0.1992125984251968684 ) ) ;
#18988=ORIENTED_EDGE ( 'NONE', *, *, #7076, .F. ) ;
#19003=CARTESIAN_POINT ( 'NONE',  ( 0.4061284506583976994, -0.2351468520617074898, 0.1992125984251968684 ) ) ;
#19006=APPLICATION_CONTEXT ( 'automotive_design' ) ;
#19009=EDGE_CURVE ( 'NONE', #9793, #5280, #6636, .T. ) ;
#19010=AXIS2_PLACEMENT_3D ( 'NONE', #19915, #23383, #567 ) ;
#19012=EDGE_CURVE ( 'NONE', #16931, #339, #19529, .T. ) ;
#19015=AXIS2_PLACEMENT_3D ( 'NONE', #24101, #11237, #8976 ) ;
#19016=CARTESIAN_POINT ( 'NONE',  ( 0.0005896702191549359900, 0.4865884552403887398, 0.1827409795202793175 ) ) ;
#19025=CARTESIAN_POINT ( 'NONE',  ( -0.3020979083623086536, 0.3591256245825952265, 0.07637795275590551769 ) ) ;
#19036=VERTEX_POINT ( 'NONE', #26810 ) ;
#19040=ORIENTED_EDGE ( 'NONE', *, *, #24013, .F. ) ;
#19069=AXIS2_PLACEMENT_3D ( 'NONE', #10285, #16244, #12130 ) ;
#19075=SPHERICAL_SURFACE ( 'NONE', #7672, 0.07677362204724409722 ) ;
#19087=TOROIDAL_SURFACE ( 'NONE', #2828, 0.4232283464566928832, 0.07677165354330708902 ) ;
#19091=CARTESIAN_POINT ( 'NONE',  ( -1.456051859514965975E-17, 0.4692913385826771866, 0.1992150590373740204 ) ) ;
#19108=DIRECTION ( 'NONE',  ( 0.000000000000000000, 0.000000000000000000, 1.000000000000000000 ) ) ;
#19124=B_SPLINE_CURVE_WITH_KNOTS ( 'NONE', 3,
 ( #20251, #7538, #11920, #26602, #3144, #9649 ),
 .UNSPECIFIED., .F., .F.,
 ( 4, 2, 4 ),
 ( 0.7157687286427140139, 0.7172350147555660582, 0.7187013008684189908 ),
 .UNSPECIFIED. ) ;
#19127=ORIENTED_EDGE ( 'NONE', *, *, #251, .F. ) ;
#19146=DIRECTION ( 'NONE',  ( 0.000000000000000000, 0.000000000000000000, 1.000000000000000000 ) ) ;
#19152=CARTESIAN_POINT ( 'NONE',  ( 0.3015429802568458384, -0.1746717017766615809, 0.1589462317943655945 ) ) ;
#19154=DIRECTION ( 'NONE',  ( -0.9396926207859082059, -0.3420201433256691015, 0.000000000000000000 ) ) ;
#19159=EDGE_CURVE ( 'NONE', #16146, #16265, #25111, .T. ) ;
#19162=ORIENTED_EDGE ( 'NONE', *, *, #9210, .F. ) ;
#19164=CARTESIAN_POINT ( 'NONE',  ( 0.000000000000000000, 0.000000000000000000, 0.2637795275590551491 ) ) ;
#19168=AXIS2_PLACEMENT_3D ( 'NONE', #1936, #4335, #2074 ) ;
#19184=AXIS2_PLACEMENT_3D ( 'NONE', #26142, #21907, #13550 ) ;
#19202=CARTESIAN_POINT ( 'NONE',  ( 0.5393700787401575214, 0.000000000000000000, 0.2755905511811023723 ) ) ;
#19221=AXIS2_PLACEMENT_3D ( 'NONE', #26996, #3520, #24864 ) ;
#19231=DIRECTION ( 'NONE',  ( 0.1736481776669301369, -0.9848077530122081313, 0.000000000000000000 ) ) ;
#19239=B_SPLINE_CURVE_WITH_KNOTS ( 'NONE', 3,
 ( #27156, #4121, #4263, #326, #10753, #3982 ),
 .UNSPECIFIED., .F., .F.,
 ( 4, 2, 4 ),
 ( 0.000000000000000000, 0.2500000000000000000, 0.5000000000000000000 ),
 .UNSPECIFIED. ) ;
#19242=ORIENTED_EDGE ( 'NONE', *, *, #11446, .F. ) ;
#19245=TOROIDAL_SURFACE ( 'NONE', #13839, 0.4232283464566928832, 0.07677165354330708902 ) ;
#19256=DIRECTION ( 'NONE',  ( 0.000000000000000000, 0.000000000000000000, 1.000000000000000000 ) ) ;
#19262=CARTESIAN_POINT ( 'NONE',  ( -0.4327133464953751840, -0.2505177833316183933, 0.1259302777263945627 ) ) ;
#19270=ORIENTED_EDGE ( 'NONE', *, *, #25719, .T. ) ;
#19296=CARTESIAN_POINT ( 'NONE',  ( 0.0005896702191646874128, 0.4865884552430826959, 0.09284957166429574915 ) ) ;
#19300=ORIENTED_EDGE ( 'NONE', *, *, #11931, .F. ) ;
#19314=CARTESIAN_POINT ( 'NONE',  ( -0.1704479274139978628, -0.4700505334955267234, 0.1496602734641385990 ) ) ;
#19317=CIRCLE ( 'NONE', #15263, 0.3771653543307086909 ) ;
#19331=B_SPLINE_CURVE_WITH_KNOTS ( 'NONE', 3,
 ( #16632, #27232, #27096, #25247, #7744, #24960 ),
 .UNSPECIFIED., .F., .F.,
 ( 4, 2, 4 ),
 ( 0.2291966065698859967, 0.2305109203526899964, 0.2318252341354939960 ),
 .UNSPECIFIED. ) ;
#19336=CARTESIAN_POINT ( 'NONE',  ( 0.3002886982018046491, -0.1727973894384566000, 0.1377952755905509363 ) ) ;
#19339=CIRCLE ( 'NONE', #15311, 0.07677362204724409722 ) ;
#19341=CARTESIAN_POINT ( 'NONE',  ( -0.4620608682196457040, 0.08206165078054665496, 0.07637795275590551769 ) ) ;
#19345=B_SPLINE_CURVE_WITH_KNOTS ( 'NONE', 3,
 ( #18334, #854, #994, #26536, #11575, #5214 ),
 .UNSPECIFIED., .F., .F.,
 ( 4, 2, 4 ),
 ( 0.5000000000000000000, 0.7500000000000000000, 1.000000000000000000 ),
 .UNSPECIFIED. ) ;
#19351=CARTESIAN_POINT ( 'NONE',  ( 0.1293227632562456708, -0.3543012242648960752, 0.07637630750536809898 ) ) ;
#19362=CARTESIAN_POINT ( 'NONE',  ( 0.3002886982018046491, -0.1727973894384566000, 0.1377952755905509363 ) ) ;
#19363=CARTESIAN_POINT ( 'NONE',  ( 0.2358179517425398330, 0.2802411498256521249, 0.1910323752979251055 ) ) ;
#19374=CARTESIAN_POINT ( 'NONE',  ( 0.2420394123212937232, 0.2892587550802425134, 0.1992125984251968684 ) ) ;
#19381=ADVANCED_FACE ( 'NONE', ( #23137 ), #11991, .F. ) ;
#19392=CARTESIAN_POINT ( 'NONE',  ( -0.2997912780622379314, -0.1736589463928940036, 0.1478915661223339784 ) ) ;
#19398=DIRECTION ( 'NONE',  ( 0.000000000000000000, 0.000000000000000000, 1.000000000000000000 ) ) ;
#19400=ADVANCED_FACE ( 'NONE', ( #3770, #14680 ), #7594, .T. ) ;
#19418=CARTESIAN_POINT ( 'NONE',  ( -0.1601448837025507554, -0.4411213145380000200, 0.07637630773773071424 ) ) ;
#19430=ADVANCED_FACE ( 'NONE', ( #1350 ), #8389, .F. ) ;
#19434=DIRECTION ( 'NONE',  ( 0.000000000000000000, 0.000000000000000000, -1.000000000000000000 ) ) ;
#19439=DIRECTION ( 'NONE',  ( 0.000000000000000000, 1.000000000000000000, 0.000000000000000000 ) ) ;
#19444=CARTESIAN_POINT ( 'NONE',  ( 0.000000000000000000, 0.000000000000000000, 0.1992125984251968684 ) ) ;
#19446=DIRECTION ( 'NONE',  ( 0.000000000000000000, 0.000000000000000000, 1.000000000000000000 ) ) ;
#19454=VERTEX_POINT ( 'NONE', #20568 ) ;
#19464=VERTEX_POINT ( 'NONE', #16329 ) ;
#19465=CARTESIAN_POINT ( 'NONE',  ( -0.1706130639253582437, -0.4670119966449340909, 0.1615162260892915869 ) ) ;
#19474=AXIS2_PLACEMENT_3D ( 'NONE', #12895, #92, #6686 ) ;
#19479=CIRCLE ( 'NONE', #17229, 0.3771653543307086909 ) ;
#19496=TOROIDAL_SURFACE ( 'NONE', #6875, 0.4232283464566928832, 0.07677165354330708902 ) ;
#19501=DIRECTION ( 'NONE',  ( 0.000000000000000000, 0.000000000000000000, 1.000000000000000000 ) ) ;
#19507=CARTESIAN_POINT ( 'NONE',  ( 0.2223167940359795647, 0.2657206863494897542, 0.1377952755905510474 ) ) ;
#19508=CARTESIAN_POINT ( 'NONE',  ( 0.4622619257814346572, 0.08092139668567618904, 0.07637795275590551769 ) ) ;
#19509=CARTESIAN_POINT ( 'NONE',  ( -0.2427018018350767803, 0.2887032559529634224, 0.07637630750536809898 ) ) ;
#19511=AXIS2_PLACEMENT_3D ( 'NONE', #23124, #19146, #6309 ) ;
#19512=CARTESIAN_POINT ( 'NONE',  ( -0.0001924259990621056968, 0.4692913385826771866, 0.1992150590373740204 ) ) ;
#19517=CARTESIAN_POINT ( 'NONE',  ( 0.1610509776512037416, -0.4407912692718771175, 0.07637795275590551769 ) ) ;
#19518=EDGE_LOOP ( 'NONE', ( #25448, #25402, #7878, #16857 ) ) ;
#19529=B_SPLINE_CURVE_WITH_KNOTS ( 'NONE', 3,
 ( #17558, #2563, #10632, #24316, #4964, #2825 ),
 .UNSPECIFIED., .F., .F.,
 ( 4, 2, 4 ),
 ( 0.6902184472752670441, 0.6915327610580700446, 0.6928470748408740443 ),
 .UNSPECIFIED. ) ;
#19532=CARTESIAN_POINT ( 'NONE',  ( 0.4621283342336283129, 0.08168108835549410529, 0.07637549214372854611 ) ) ;
#19537=SURFACE_SIDE_STYLE ('',( #24187 ) ) ;
#19571=CIRCLE ( 'NONE', #7375, 0.3771653543307086909 ) ;
#19573=EDGE_CURVE ( 'NONE', #26656, #18025, #20875, .T. ) ;
#19578=TOROIDAL_SURFACE ( 'NONE', #19511, 0.4232283464566928832, 0.07677165354330708902 ) ;
#19595=EDGE_CURVE ( 'NONE', #19464, #21723, #20101, .T. ) ;
#19604=DIRECTION ( 'NONE',  ( 0.000000000000000000, 0.000000000000000000, 1.000000000000000000 ) ) ;
#19610=ORIENTED_EDGE ( 'NONE', *, *, #21879, .F. ) ;
#19622=ORIENTED_EDGE ( 'NONE', *, *, #21879, .T. ) ;
#19629=ORIENTED_EDGE ( 'NONE', *, *, #1371, .T. ) ;
#19636=CIRCLE ( 'NONE', #20974, 0.3464566929133857665 ) ;
#19637=CARTESIAN_POINT ( 'NONE',  ( -0.2720459371704843088, 0.3242117229735834716, 0.1377952755905511861 ) ) ;
#19638=VERTEX_POINT ( 'NONE', #16895 ) ;
#19639=CARTESIAN_POINT ( 'NONE',  ( -0.4897507849286801829, 0.08575075074550207732, 0.1615162260910394110 ) ) ;
#19641=CARTESIAN_POINT ( 'NONE',  ( -0.3528204557975102018, 0.06272520244122334332, 0.09506557083631544947 ) ) ;
#19646=AXIS2_PLACEMENT_3D ( 'NONE', #18598, #27527, #1663 ) ;
#19653=CARTESIAN_POINT ( 'NONE',  ( 0.000000000000000000, 0.000000000000000000, 0.1992125984251968684 ) ) ;
#19665=DIRECTION ( 'NONE',  ( 0.000000000000000000, 0.000000000000000000, -1.000000000000000000 ) ) ;
#19669=ORIENTED_EDGE ( 'NONE', *, *, #17363, .F. ) ;
#19688=DIRECTION ( 'NONE',  ( 0.000000000000000000, 0.000000000000000000, 1.000000000000000000 ) ) ;
#19713=AXIS2_PLACEMENT_3D ( 'NONE', #23598, #21874, #13948 ) ;
#19724=CARTESIAN_POINT ( 'NONE',  ( -0.1294857240059045234, -0.3542416573274181357, 0.1992125984251968684 ) ) ;
#19727=FACE_OUTER_BOUND ( 'NONE', #5629, .T. ) ;
#19738=ORIENTED_EDGE ( 'NONE', *, *, #10013, .T. ) ;
#19760=CARTESIAN_POINT ( 'NONE',  ( 0.4211031283173693462, -0.2438048970101359125, 0.09284957166162138842 ) ) ;
#19770=AXIS2_PLACEMENT_3D ( 'NONE', #2819, #20209, #729 ) ;
#19791=B_SPLINE_CURVE_WITH_KNOTS ( 'NONE', 3,
 ( #25387, #6, #23701, #6597, #27522, #18875 ),
 .UNSPECIFIED., .F., .F.,
 ( 4, 2, 4 ),
 ( 0.000000000000000000, 0.2500000000000000000, 0.5000000000000000000 ),
 .UNSPECIFIED. ) ;
#19803=EDGE_LOOP ( 'NONE', ( #21372, #25122, #21927, #4211 ) ) ;
#19809=CARTESIAN_POINT ( 'NONE',  ( -0.2720459371704843088, 0.3242117229735834716, 0.06102165354330708891 ) ) ;
#19812=VERTEX_POINT ( 'NONE', #5268 ) ;
#19820=AXIS2_PLACEMENT_3D ( 'NONE', #13441, #6798, #17253 ) ;
#19847=AXIS2_PLACEMENT_3D ( 'NONE', #16969, #1566, #25297 ) ;
#19863=ORIENTED_EDGE ( 'NONE', *, *, #13706, .T. ) ;
#19876=VERTEX_POINT ( 'NONE', #5119 ) ;
#19891=DIRECTION ( 'NONE',  ( -1.000000000000000000, 1.224646799147353454E-16, 0.000000000000000000 ) ) ;
#19898=DIRECTION ( 'NONE',  ( 0.000000000000000000, 1.000000000000000000, 0.000000000000000000 ) ) ;
#19903=CARTESIAN_POINT ( 'NONE',  ( -0.4061284506584276199, -0.2351468520616558922, 0.07637795275590551769 ) ) ;
#19907=CARTESIAN_POINT ( 'NONE',  ( 0.000000000000000000, 0.000000000000000000, 0.01181102362204724393 ) ) ;
#19908=CARTESIAN_POINT ( 'NONE',  ( -0.3411065095061436847, 0.06065137456822528028, 0.1276989850548526373 ) ) ;
#19915=CARTESIAN_POINT ( 'NONE',  ( 0.000000000000000000, 0.000000000000000000, 0.07637795275590551769 ) ) ;
#19916=DIRECTION ( 'NONE',  ( 0.000000000000000000, -1.000000000000000000, 0.000000000000000000 ) ) ;
#19933=VERTEX_POINT ( 'NONE', #8240 ) ;
#19943=CIRCLE ( 'NONE', #24441, 0.3771653543307086909 ) ;
#19946=CYLINDRICAL_SURFACE ( 'NONE', #5839, 0.3771653543307086909 ) ;
#19956=CARTESIAN_POINT ( 'NONE',  ( 0.0005056364805201059732, 0.3583524373864921952, 0.1805249803418951804 ) ) ;
#19959=AXIS2_PLACEMENT_3D ( 'NONE', #22631, #3253, #5542 ) ;
#19971=AXIS2_PLACEMENT_3D ( 'NONE', #21088, #12748, #1593 ) ;
#19975=CARTESIAN_POINT ( 'NONE',  ( -3.616083068348483797E-17, -0.2952755905511810774, 0.2637795275590551491 ) ) ;
#19985=ORIENTED_EDGE ( 'NONE', *, *, #26961, .F. ) ;
#19997=EDGE_LOOP ( 'NONE', ( #26991, #26131, #4374, #18322 ) ) ;
#20022=CIRCLE ( 'NONE', #11450, 0.01181102362204724046 ) ;
#20025=CARTESIAN_POINT ( 'NONE',  ( 0.000000000000000000, 0.000000000000000000, 0.07637795275590551769 ) ) ;
#20037=ORIENTED_EDGE ( 'NONE', *, *, #2917, .F. ) ;
#20061=CARTESIAN_POINT ( 'NONE',  ( -0.3082037322256093170, 0.3663931537939284500, 0.1920935997048431876 ) ) ;
#20066=CARTESIAN_POINT ( 'NONE',  ( -0.1293227632562458651, -0.3543012242648960752, 0.07637630750536809898 ) ) ;
#20074=EDGE_LOOP ( 'NONE', ( #22800, #26923, #22163, #19863, #25575, #803, #6212, #22584, #14491, #10916, #14691, #4378, #10447, #26805 ) ) ;
#20075=B_SPLINE_CURVE_WITH_KNOTS ( 'NONE', 3,
 ( #11609, #20230, #890, #9621, #16143, #24740 ),
 .UNSPECIFIED., .F., .F.,
 ( 4, 2, 4 ),
 ( 0.2291966065698869959, 0.2305109203526899964, 0.2318252341354939960 ),
 .UNSPECIFIED. ) ;
#20092=CARTESIAN_POINT ( 'NONE',  ( 0.0004974201395668345887, 0.3464563358313496044, 0.1478915661244618873 ) ) ;
#20094=CARTESIAN_POINT ( 'NONE',  ( 0.3218517393631780688, 0.3826375019114283682, 0.1259302777232058079 ) ) ;
#20095=B_SPLINE_CURVE_WITH_KNOTS ( 'NONE', 3,
 ( #1392, #8050, #8184, #10012, #25832, #10566 ),
 .UNSPECIFIED., .F., .F.,
 ( 4, 2, 4 ),
 ( 0.000000000000000000, 0.2500000000000000000, 0.5000000000000000000 ),
 .UNSPECIFIED. ) ;
#20101=CIRCLE ( 'NONE', #27333, 0.3464566929133857665 ) ;
#20108=ORIENTED_EDGE ( 'NONE', *, *, #11834, .T. ) ;
#20121=CARTESIAN_POINT ( 'NONE',  ( -5.747161356628524594E-17, -0.4692913385826771866, 0.07637795275590551769 ) ) ;
#20143=ORIENTED_EDGE ( 'NONE', *, *, #14676, .F. ) ;
#20153=DIRECTION ( 'NONE',  ( 0.000000000000000000, 0.000000000000000000, 1.000000000000000000 ) ) ;
#20154=CIRCLE ( 'NONE', #15710, 0.5511811023622047445 ) ;
#20156=AXIS2_PLACEMENT_3D ( 'NONE', #26216, #19446, #25948 ) ;
#20170=CARTESIAN_POINT ( 'NONE',  ( -0.4925073816775267788, 0.08623502184948558802, 0.1259302777239357518 ) ) ;
#20175=CARTESIAN_POINT ( 'NONE',  ( -0.3430989538742943989, 0.06100393589344793588, 0.1166443193847512133 ) ) ;
#20180=VERTEX_POINT ( 'NONE', #26292 ) ;
#20183=CARTESIAN_POINT ( 'NONE',  ( 0.1294857240059045234, -0.3542416573274181357, 0.07637795275590551769 ) ) ;
#20187=DIRECTION ( 'NONE',  ( 1.000000000000000000, 0.000000000000000000, 0.000000000000000000 ) ) ;
#20189=DIRECTION ( 'NONE',  ( 0.000000000000000000, 0.000000000000000000, 1.000000000000000000 ) ) ;
#20207=EDGE_CURVE ( 'NONE', #23369, #9720, #3408, .T. ) ;
#20209=DIRECTION ( 'NONE',  ( 0.000000000000000000, 0.000000000000000000, 1.000000000000000000 ) ) ;
#20219=CIRCLE ( 'NONE', #5802, 0.4692913385826771866 ) ;
#20229=EDGE_CURVE ( 'NONE', #27155, #12220, #21532, .T. ) ;
#20230=CARTESIAN_POINT ( 'NONE',  ( -0.3714952424334504455, 0.06515381386493838967, 0.07637630750536809898 ) ) ;
#20232=CARTESIAN_POINT ( 'NONE',  ( 0.1220886091274603069, -0.3369140789169591255, 0.09506557083486352755 ) ) ;
#20251=CARTESIAN_POINT ( 'NONE',  ( -0.1599629598573265865, -0.4411872753632007926, 0.1992125984251968684 ) ) ;
#20258=DIRECTION ( 'NONE',  ( 0.000000000000000000, 0.000000000000000000, 1.000000000000000000 ) ) ;
#20264=EDGE_CURVE ( 'NONE', #3213, #23387, #7016, .T. ) ;
#20285=ORIENTED_EDGE ( 'NONE', *, *, #18141, .T. ) ;
#20297=DIRECTION ( 'NONE',  ( 0.3420201433256691015, -0.9396926207859082059, 0.000000000000000000 ) ) ;
#20302=CARTESIAN_POINT ( 'NONE',  ( -0.4067073728345788064, -0.2341441294389334793, 0.1992125984251968684 ) ) ;
#20305=CARTESIAN_POINT ( 'NONE',  ( 0.1599629598573824862, -0.4411872753631803090, 0.07637795275590551769 ) ) ;
#20323=ORIENTED_EDGE ( 'NONE', *, *, #18548, .T. ) ;
#20330=B_SPLINE_CURVE_WITH_KNOTS ( 'NONE', 3,
 ( #10630, #27459, #14632, #3560, #12192, #20814 ),
 .UNSPECIFIED., .F., .F.,
 ( 4, 2, 4 ),
 ( 0.2376120521391529850, 0.2390783382518550104, 0.2405446243645580073 ),
 .UNSPECIFIED. ) ;
#20352=AXIS2_PLACEMENT_3D ( 'NONE', #5772, #1518, #3775 ) ;
#20357=DIRECTION ( 'NONE',  ( 0.000000000000000000, -1.000000000000000000, 0.000000000000000000 ) ) ;
#20370=FACE_OUTER_BOUND ( 'NONE', #7799, .T. ) ;
#20373=EDGE_CURVE ( 'NONE', #935, #16738, #18395, .T. ) ;
#20378=CIRCLE ( 'NONE', #25814, 0.2952755905511810774 ) ;
#20407=TOROIDAL_SURFACE ( 'NONE', #27646, 0.4232283464566928832, 0.07677165354330708902 ) ;
#20408=ADVANCED_FACE ( 'NONE', ( #4957 ), #22190, .F. ) ;
#20412=CARTESIAN_POINT ( 'NONE',  ( 0.000000000000000000, 0.000000000000000000, 0.1377952755905511861 ) ) ;
#20415=FACE_OUTER_BOUND ( 'NONE', #18566, .T. ) ;
#20418=EDGE_LOOP ( 'NONE', ( #26946, #10825, #22406, #20922 ) ) ;
#20423=ORIENTED_EDGE ( 'NONE', *, *, #23246, .F. ) ;
#20425=AXIS2_PLACEMENT_3D ( 'NONE', #16845, #4267, #6384 ) ;
#20427=CARTESIAN_POINT ( 'NONE',  ( 0.0005189969344232283309, 0.3771649972486724733, 0.1992125984251968684 ) ) ;
#20468=ORIENTED_EDGE ( 'NONE', *, *, #15081, .T. ) ;
#20471=FACE_OUTER_BOUND ( 'NONE', #12188, .T. ) ;
#20496=ORIENTED_EDGE ( 'NONE', *, *, #20889, .F. ) ;
#20535=ORIENTED_EDGE ( 'NONE', *, *, #23347, .T. ) ;
#20541=DIRECTION ( 'NONE',  ( 1.000000000000000000, 0.000000000000000000, 0.000000000000000000 ) ) ;
#20561=ORIENTED_EDGE ( 'NONE', *, *, #11302, .T. ) ;
#20563=ORIENTED_EDGE ( 'NONE', *, *, #2477, .F. ) ;
#20568=CARTESIAN_POINT ( 'NONE',  ( -0.3713448905834433322, 0.06600512665679449109, 0.07637795275590551769 ) ) ;
#20580=B_SPLINE_CURVE_WITH_KNOTS ( 'NONE', 3,
 ( #4779, #2384, #555, #2658, #20170, #9280, #19639, #21754, #17892, #22293 ),
 .UNSPECIFIED., .F., .F.,
 ( 4, 2, 2, 2, 4 ),
 ( 0.000000000000000000, 0.2500000000000000000, 0.5000000000000000000, 0.7500000000000000000, 1.000000000000000000 ),
 .UNSPECIFIED. ) ;
#20597=AXIS2_PLACEMENT_3D ( 'NONE', #15293, #4535, #17117 ) ;
#20600=ORIENTED_EDGE ( 'NONE', *, *, #26972, .T. ) ;
#20602=DIRECTION ( 'NONE',  ( 1.000000000000000000, 0.000000000000000000, 0.000000000000000000 ) ) ;
#20608=ORIENTED_EDGE ( 'NONE', *, *, #17104, .F. ) ;
#20610=ORIENTED_EDGE ( 'NONE', *, *, #10132, .T. ) ;
#20614=CARTESIAN_POINT ( 'NONE',  ( 0.000000000000000000, 0.000000000000000000, 0.1377952755905511861 ) ) ;
#20619=AXIS2_PLACEMENT_3D ( 'NONE', #24902, #22511, #18248 ) ;
#20628=CARTESIAN_POINT ( 'NONE',  ( -0.2299571666332044795, 0.2748389101983655380, 0.09506557084787936596 ) ) ;
#20648=CIRCLE ( 'NONE', #8474, 0.3771653543307086909 ) ;
#20652=DIRECTION ( 'NONE',  ( -0.3420201433256691015, -0.9396926207859082059, 0.000000000000000000 ) ) ;
#20655=CARTESIAN_POINT ( 'NONE',  ( -0.1294857240059045234, -0.3542416573274181357, 0.1992125984251968684 ) ) ;
#20680=CARTESIAN_POINT ( 'NONE',  ( -0.2236164729188093725, 0.2672714825438527453, 0.1589462317847418760 ) ) ;
#20710=TOROIDAL_SURFACE ( 'NONE', #12590, 0.4232283464566928832, 0.07677165354330708902 ) ;
#20722=DIRECTION ( 'NONE',  ( 1.000000000000000000, 0.000000000000000000, 0.000000000000000000 ) ) ;
#20727=VERTEX_POINT ( 'NONE', #13273 ) ;
#20734=B_SPLINE_CURVE_WITH_KNOTS ( 'NONE', 3,
 ( #18657, #12603, #14757, #21224, #1306, #20794 ),
 .UNSPECIFIED., .F., .F.,
 ( 4, 2, 4 ),
 ( 0.6902184472752670441, 0.6915327610580710438, 0.6928470748408740443 ),
 .UNSPECIFIED. ) ;
#20758=DIRECTION ( 'NONE',  ( -0.4999999999999995004, 0.8660254037844390407, 0.000000000000000000 ) ) ;
#20759=CIRCLE ( 'NONE', #19847, 0.5511811023622047445 ) ;
#20763=SPHERICAL_SURFACE ( 'NONE', #16414, 0.07677362204724409722 ) ;
#20765=CARTESIAN_POINT ( 'NONE',  ( 0.5511811023622047445, 0.000000000000000000, 0.01181102362204724393 ) ) ;
#20775=ORIENTED_EDGE ( 'NONE', *, *, #25343, .F. ) ;
#20794=CARTESIAN_POINT ( 'NONE',  ( 0.2420394123212937232, 0.2892587550802425134, 0.1992125984251968684 ) ) ;
#20798=EDGE_CURVE ( 'NONE', #2204, #27155, #16411, .T. ) ;
#20814=CARTESIAN_POINT ( 'NONE',  ( 0.3012109481302311376, 0.3598698725862007897, 0.07637795275590551769 ) ) ;
#20842=AXIS2_PLACEMENT_3D ( 'NONE', #6274, #8522, #8792 ) ;
#20846=DIRECTION ( 'NONE',  ( 0.1736481776669300814, -0.9848077530122080203, 0.000000000000000000 ) ) ;
#20848=EDGE_LOOP ( 'NONE', ( #20496, #6211 ) ) ;
#20851=AXIS2_PLACEMENT_3D ( 'NONE', #15329, #26174, #12307 ) ;
#20875=B_SPLINE_CURVE_WITH_KNOTS ( 'NONE', 3,
 ( #7997, #5882, #25076, #23112, #21124, #14511 ),
 .UNSPECIFIED., .F., .F.,
 ( 4, 2, 4 ),
 ( 0.7157687286427140139, 0.7172350147555670574, 0.7187013008684189908 ),
 .UNSPECIFIED. ) ;
#20876=VERTEX_POINT ( 'NONE', #21966 ) ;
#20882=VERTEX_POINT ( 'NONE', #15617 ) ;
#20883=ORIENTED_EDGE ( 'NONE', *, *, #15702, .T. ) ;
#20889=EDGE_CURVE ( 'NONE', #10900, #17397, #23425, .T. ) ;
#20894=CARTESIAN_POINT ( 'NONE',  ( -0.2428345617565149384, 0.2885915454824177218, 0.1992125984251968684 ) ) ;
#20898=VERTEX_POINT ( 'NONE', #19975 ) ;
#20903=DIRECTION ( 'NONE',  ( 1.000000000000000000, 0.000000000000000000, 0.000000000000000000 ) ) ;
#20913=CARTESIAN_POINT ( 'NONE',  ( 0.000000000000000000, 0.000000000000000000, 0.1377952755905511861 ) ) ;
#20921=FACE_OUTER_BOUND ( 'NONE', #19518, .T. ) ;
#20922=ORIENTED_EDGE ( 'NONE', *, *, #16818, .T. ) ;
#20926=CARTESIAN_POINT ( 'NONE',  ( -0.4167985568850881561, 0.07349283109919312051, 0.2145688976377952695 ) ) ;
#20930=ORIENTED_EDGE ( 'NONE', *, *, #20373, .T. ) ;
#20955=EDGE_CURVE ( 'NONE', #16432, #15505, #10011, .T. ) ;
#20973=ORIENTED_EDGE ( 'NONE', *, *, #27826, .T. ) ;
#20974=AXIS2_PLACEMENT_3D ( 'NONE', #17588, #2470, #15363 ) ;
#20979=CARTESIAN_POINT ( 'NONE',  ( 0.000000000000000000, 0.000000000000000000, 0.1992125984251968684 ) ) ;
#21003=CARTESIAN_POINT ( 'NONE',  ( 0.3123213164519275664, 0.3731274149352674097, 0.09284957166392941719 ) ) ;
#21008=CARTESIAN_POINT ( 'NONE',  ( -0.4620608682196346573, 0.08206165078060512208, 0.1992125984251968684 ) ) ;
#21015=CARTESIAN_POINT ( 'NONE',  ( -0.1294857240059045234, -0.3542416573274181357, 0.07637795275590551769 ) ) ;
#21021=CARTESIAN_POINT ( 'NONE',  ( -0.0005189969344232283309, 0.3771649972486724733, 0.07637795275590551769 ) ) ;
#21075=EDGE_CURVE ( 'NONE', #17199, #19638, #2249, .T. ) ;
#21081=EDGE_CURVE ( 'NONE', #22192, #26883, #26170, .T. ) ;
#21088=CARTESIAN_POINT ( 'NONE',  ( 0.000000000000000000, 0.000000000000000000, 0.1992125984251968684 ) ) ;
#21103=EDGE_CURVE ( 'NONE', #24815, #16432, #23831, .T. ) ;
#21110=CARTESIAN_POINT ( 'NONE',  ( 0.3073078020556853085, 0.3671449284689711212, 0.1920935997049015298 ) ) ;
#21116=CARTESIAN_POINT ( 'NONE',  ( -0.5511811023622047445, 6.750021727583836750E-17, 0.2637795275590551491 ) ) ;
#21124=CARTESIAN_POINT ( 'NONE',  ( 0.3019498226894488102, 0.3592501948414881796, 0.1992142434433716580 ) ) ;
#21134=CARTESIAN_POINT ( 'NONE',  ( 0.3263749705684267921, -0.1890319631540330891, 0.07637795275590551769 ) ) ;
#21136=AXIS2_PLACEMENT_3D ( 'NONE', #9202, #7376, #13589 ) ;
#21142=CARTESIAN_POINT ( 'NONE',  ( 0.0005963271530293720634, 0.4972008316414386897, 0.1615162260929392524 ) ) ;
#21144=DIRECTION ( 'NONE',  ( 0.000000000000000000, 0.000000000000000000, 1.000000000000000000 ) ) ;
#21152=DIRECTION ( 'NONE',  ( 0.000000000000000000, 1.000000000000000000, 0.000000000000000000 ) ) ;
#21154=CARTESIAN_POINT ( 'NONE',  ( -0.3018020646414484309, 0.3593743330771480560, 0.07637549214372835182 ) ) ;
#21167=ORIENTED_EDGE ( 'NONE', *, *, #23983, .F. ) ;
#21179=CARTESIAN_POINT ( 'NONE',  ( 0.2223167940359795647, 0.2657206863494897542, 0.1377952755905510474 ) ) ;
#21194=EDGE_CURVE ( 'NONE', #1637, #8715, #429, .T. ) ;
#21197=CARTESIAN_POINT ( 'NONE',  ( -0.1447526197146041249, -0.3977045540727763839, 0.06102165354330708891 ) ) ;
#21224=CARTESIAN_POINT ( 'NONE',  ( 0.2423050875943940918, 0.2890362931940642088, 0.1992150590373740204 ) ) ;
#21231=VERTEX_POINT ( 'NONE', #12893 ) ;
#21238=CARTESIAN_POINT ( 'NONE',  ( 0.000000000000000000, 0.000000000000000000, 0.1377952755905511584 ) ) ;
#21241=ADVANCED_FACE ( 'NONE', ( #17675 ), #15451, .F. ) ;
#21255=CARTESIAN_POINT ( 'NONE',  ( -0.3020979083623086536, 0.3591256245825952265, 0.07637795275590551769 ) ) ;
#21302=VERTEX_POINT ( 'NONE', #25896 ) ;
#21304=ORIENTED_EDGE ( 'NONE', *, *, #10132, .F. ) ;
#21329=MANIFOLD_SOLID_BREP ( 'Deep Groove Ball Bearing 15x28x7', #25875 ) ;
#21334=CARTESIAN_POINT ( 'NONE',  ( -0.4620947063919693121, 0.08187111969648680487, 0.07637630773773071424 ) ) ;
#21339=VERTEX_POINT ( 'NONE', #7651 ) ;
#21351=PLANE ( 'NONE',  #21766 ) ;
#21356=CARTESIAN_POINT ( 'NONE',  ( 0.2223167940359795092, 0.2657206863494898097, 0.1478915661212649724 ) ) ;
#21372=ORIENTED_EDGE ( 'NONE', *, *, #14581, .T. ) ;
#21378=CIRCLE ( 'NONE', #9612, 0.3771653543307086909 ) ;
#21417=B_SPLINE_CURVE_WITH_KNOTS ( 'NONE', 3,
 ( #17245, #4531, #13135, #21765, #7472, #986 ),
 .UNSPECIFIED., .F., .F.,
 ( 4, 2, 4 ),
 ( 0.000000000000000000, 0.2500000000000000000, 0.5000000000000000000 ),
 .UNSPECIFIED. ) ;
#21447=CARTESIAN_POINT ( 'NONE',  ( -0.1632039128461710842, -0.4501088385475445208, 0.08349695147787532246 ) ) ;
#21464=CARTESIAN_POINT ( 'NONE',  ( 0.4620608682196457040, 0.08206165078054626638, 0.07637795275590551769 ) ) ;
#21474=EDGE_CURVE ( 'NONE', #27620, #10277, #12262, .T. ) ;
#21480=AXIS2_PLACEMENT_3D ( 'NONE', #24071, #4707, #2583 ) ;
#21486=VERTEX_POINT ( 'NONE', #6108 ) ;
#21487=CARTESIAN_POINT ( 'NONE',  ( 0.3002886982018043160, -0.1727973894384573772, 0.1276989850532580795 ) ) ;
#21491=DIRECTION ( 'NONE',  ( 0.000000000000000000, 0.000000000000000000, 1.000000000000000000 ) ) ;
#21496=DIRECTION ( 'NONE',  ( -0.9396926207859082059, -0.3420201433256691015, 0.000000000000000000 ) ) ;
#21498=DIRECTION ( 'NONE',  ( 0.000000000000000000, 0.000000000000000000, -1.000000000000000000 ) ) ;
#21510=AXIS2_PLACEMENT_3D ( 'NONE', #8486, #17108, #23085 ) ;
#21512=ORIENTED_EDGE ( 'NONE', *, *, #14788, .F. ) ;
#21529=CARTESIAN_POINT ( 'NONE',  ( -0.4143458349576718547, -0.2398979215369355655, 0.1920935997051132493 ) ) ;
#21532=B_SPLINE_CURVE_WITH_KNOTS ( 'NONE', 3,
 ( #6816, #23781, #4422, #23510, #23918, #2011 ),
 .UNSPECIFIED., .F., .F.,
 ( 4, 2, 4 ),
 ( 0.000000000000000000, 0.2500000000000000000, 0.5000000000000000000 ),
 .UNSPECIFIED. ) ;
#21534=CARTESIAN_POINT ( 'NONE',  ( 0.1643029338967702813, -0.4497088275954951309, 0.1920935997051998190 ) ) ;
#21559=CARTESIAN_POINT ( 'NONE',  ( 0.0005789221761808661720, 0.4692909815006409691, 0.1992125984251968684 ) ) ;
#21564=CARTESIAN_POINT ( 'NONE',  ( 0.2720459371704843088, 0.3242117229735830830, 0.1377952755905511861 ) ) ;
#21595=CARTESIAN_POINT ( 'NONE',  ( 0.3020979083623086536, 0.3591256245825952265, 0.1992125984251968684 ) ) ;
#21603=EDGE_CURVE ( 'NONE', #24639, #764, #12998, .T. ) ;
#21614=EDGE_LOOP ( 'NONE', ( #7847, #24379 ) ) ;
#21631=CARTESIAN_POINT ( 'NONE',  ( 0.000000000000000000, 0.000000000000000000, 0.01181102362204724393 ) ) ;
#21633=EDGE_CURVE ( 'NONE', #15505, #24639, #21417, .T. ) ;
#21634=DIRECTION ( 'NONE',  ( 0.000000000000000000, 1.000000000000000000, 0.000000000000000000 ) ) ;
#21642=B_SPLINE_CURVE_WITH_KNOTS ( 'NONE', 3,
 ( #8217, #8360, #27149, #5677, #16692, #14297, #1424, #16534, #10040, #23054 ),
 .UNSPECIFIED., .F., .F.,
 ( 4, 2, 2, 2, 4 ),
 ( 0.000000000000000000, 0.2499999999999998335, 0.4999999999999996669, 0.7499999999999997780, 1.000000000000000000 ),
 .UNSPECIFIED. ) ;
#21645=ORIENTED_EDGE ( 'NONE', *, *, #5625, .F. ) ;
#21654=CARTESIAN_POINT ( 'NONE',  ( 0.000000000000000000, 0.000000000000000000, -3.278217716535432842E-17 ) ) ;
#21657=VERTEX_POINT ( 'NONE', #11296 ) ;
#21689=CARTESIAN_POINT ( 'NONE',  ( -0.0003454908279975297527, 0.3771652360013086902, 0.1992142436757342316 ) ) ;
#21695=FACE_OUTER_BOUND ( 'NONE', #9423, .T. ) ;
#21698=EDGE_CURVE ( 'NONE', #12220, #17730, #18374, .T. ) ;
#21708=VERTEX_POINT ( 'NONE', #4787 ) ;
#21723=VERTEX_POINT ( 'NONE', #24419 ) ;
#21730=CARTESIAN_POINT ( 'NONE',  ( -0.1643029338971332409, -0.4497088275964746806, 0.08349695147668606543 ) ) ;
#21733=B_SPLINE_CURVE_WITH_KNOTS ( 'NONE', 3,
 ( #13415, #2677, #5514, #22316 ),
 .UNSPECIFIED., .F., .F.,
 ( 4, 4 ),
 ( 0.2305109203526903294, 0.2318252341354939960 ),
 .UNSPECIFIED. ) ;
#21746=CARTESIAN_POINT ( 'NONE',  ( -0.0001924259990424426062, 0.4692913385826772976, 0.07637549214372836570 ) ) ;
#21754=CARTESIAN_POINT ( 'NONE',  ( -0.4792984784067314541, 0.08391448672285535537, 0.1827409795192550812 ) ) ;
#21765=CARTESIAN_POINT ( 'NONE',  ( 0.2243804351505061800, 0.2666304421188489537, 0.1166443193913617588 ) ) ;
#21766=AXIS2_PLACEMENT_3D ( 'NONE', #10460, #27715, #23623 ) ;
#21768=DIRECTION ( 'NONE',  ( 0.000000000000000000, 0.000000000000000000, -1.000000000000000000 ) ) ;
#21769=CARTESIAN_POINT ( 'NONE',  ( -0.0005789221761214173069, 0.4692909815006417462, 0.07637795275590551769 ) ) ;
#21787=CARTESIAN_POINT ( 'NONE',  ( 0.3411065095061437402, 0.06065137456822566192, 0.1377952755905510474 ) ) ;
#21789=CARTESIAN_POINT ( 'NONE',  ( -0.2358179517456306662, 0.2802411498293116421, 0.1910323753015176762 ) ) ;
#21832=ADVANCED_FACE ( 'NONE', ( #19727 ), #8712, .T. ) ;
#21840=DIRECTION ( 'NONE',  ( -0.9396926207859082059, 0.3420201433256691015, 0.000000000000000000 ) ) ;
#21855=CARTESIAN_POINT ( 'NONE',  ( 0.000000000000000000, 0.4692913385826771866, 0.03818897637795275884 ) ) ;
#21858=ORIENTED_EDGE ( 'NONE', *, *, #13683, .F. ) ;
#21862=CARTESIAN_POINT ( 'NONE',  ( 0.3268939675028499914, -0.1881330340946397728, 0.1992125984251968684 ) ) ;
#21867=CARTESIAN_POINT ( 'NONE',  ( -0.1610509776512594748, -0.4407912692718567449, 0.1992125984251968684 ) ) ;
#21868=CIRCLE ( 'NONE', #7005, 0.01181102362204724046 ) ;
#21873=ORIENTED_EDGE ( 'NONE', *, *, #5090, .T. ) ;
#21874=DIRECTION ( 'NONE',  ( 0.000000000000000000, 0.000000000000000000, 1.000000000000000000 ) ) ;
#21879=EDGE_CURVE ( 'NONE', #19812, #12596, #27169, .T. ) ;
#21895=DIRECTION ( 'NONE',  ( 0.000000000000000000, 0.000000000000000000, -1.000000000000000000 ) ) ;
#21901=CARTESIAN_POINT ( 'NONE',  ( 0.3606049308157521227, 0.06410376196636191626, 0.1910323753053202456 ) ) ;
#21907=DIRECTION ( 'NONE',  ( 0.9848077530122081313, 0.1736481776669301369, -0.000000000000000000 ) ) ;
#21911=CARTESIAN_POINT ( 'NONE',  ( 0.4925073816753560152, 0.08623502184910394885, 0.1259302777096748815 ) ) ;
#21914=EDGE_CURVE ( 'NONE', #5544, #10703, #14529, .T. ) ;
#21920=EDGE_LOOP ( 'NONE', ( #17161, #6395, #15415, #18138 ) ) ;
#21923=AXIS2_PLACEMENT_3D ( 'NONE', #8816, #17431, #366 ) ;
#21925=ADVANCED_FACE ( 'NONE', ( #20415 ), #2746, .F. ) ;
#21927=ORIENTED_EDGE ( 'NONE', *, *, #24777, .T. ) ;
#21930=CARTESIAN_POINT ( 'NONE',  ( 0.4620947063919693121, 0.08187111969648641630, 0.07637630773773071424 ) ) ;
#21934=CARTESIAN_POINT ( 'NONE',  ( -4.618943439303797186E-17, -0.3771653543307086909, 0.07637795275590551769 ) ) ;
#21937=DIRECTION ( 'NONE',  ( 0.000000000000000000, 0.000000000000000000, 1.000000000000000000 ) ) ;
#21941=CARTESIAN_POINT ( 'NONE',  ( 0.000000000000000000, 0.000000000000000000, 0.1377952755905511861 ) ) ;
#21948=ORIENTED_EDGE ( 'NONE', *, *, #16459, .F. ) ;
#21958=CARTESIAN_POINT ( 'NONE',  ( -0.4790936880892668892, 0.08507591033002856462, 0.1827409795186053509 ) ) ;
#21966=CARTESIAN_POINT ( 'NONE',  ( -4.618943439303797186E-17, -0.3771653543307086909, -3.278217716535432842E-17 ) ) ;
#21985=CARTESIAN_POINT ( 'NONE',  ( 0.3412792617076850221, 0.05967164814832588010, 0.1377952755905512139 ) ) ;
#21991=DIRECTION ( 'NONE',  ( -0.4999999999999995004, -0.8660254037844390407, 0.000000000000000000 ) ) ;
#21997=CARTESIAN_POINT ( 'NONE',  ( 0.3265485372158890010, -0.1887320510662011952, 0.1992150590373740204 ) ) ;
#22021=CARTESIAN_POINT ( 'NONE',  ( 0.4327133464945798758, -0.2505177833311500457, 0.1259302777204239776 ) ) ;
#22027=DIRECTION ( 'NONE',  ( 0.000000000000000000, -1.000000000000000000, 0.000000000000000000 ) ) ;
#22030=ORIENTED_EDGE ( 'NONE', *, *, #6126, .T. ) ;
#22036=FACE_OUTER_BOUND ( 'NONE', #20074, .T. ) ;
#22056=CARTESIAN_POINT ( 'NONE',  ( 0.000000000000000000, 0.000000000000000000, 0.01181102362204724393 ) ) ;
#22102=ORIENTED_EDGE ( 'NONE', *, *, #25291, .T. ) ;
#22117=DIRECTION ( 'NONE',  ( 0.000000000000000000, 1.000000000000000000, 0.000000000000000000 ) ) ;
#22126=ORIENTED_EDGE ( 'NONE', *, *, #21698, .T. ) ;
#22135=EDGE_CURVE ( 'NONE', #1348, #13865, #4882, .T. ) ;
#22145=DIRECTION ( 'NONE',  ( 0.000000000000000000, 0.000000000000000000, 1.000000000000000000 ) ) ;
#22157=ORIENTED_EDGE ( 'NONE', *, *, #23162, .T. ) ;
#22163=ORIENTED_EDGE ( 'NONE', *, *, #7834, .T. ) ;
#22171=FACE_OUTER_BOUND ( 'NONE', #19997, .T. ) ;
#22172=DIRECTION ( 'NONE',  ( 0.000000000000000000, 0.000000000000000000, 1.000000000000000000 ) ) ;
#22183=FACE_OUTER_BOUND ( 'NONE', #13669, .T. ) ;
#22186=CARTESIAN_POINT ( 'NONE',  ( 0.000000000000000000, 0.000000000000000000, 0.1992125984251968684 ) ) ;
#22187=EDGE_LOOP ( 'NONE', ( #17234, #2488, #25031, #6462 ) ) ;
#22190=CYLINDRICAL_SURFACE ( 'NONE', #19770, 0.2952755905511810774 ) ;
#22192=VERTEX_POINT ( 'NONE', #6983 ) ;
#22226=ORIENTED_EDGE ( 'NONE', *, *, #20798, .F. ) ;
#22237=CARTESIAN_POINT ( 'NONE',  ( 0.3715251363271980245, 0.06498290224717499786, 0.07637795275590551769 ) ) ;
#22245=CIRCLE ( 'NONE', #24471, 0.07677362204724409722 ) ;
#22256=EDGE_CURVE ( 'NONE', #22736, #26931, #7525, .T. ) ;
#22266=EDGE_LOOP ( 'NONE', ( #9131, #6343, #1811, #8414, #11523 ) ) ;
#22270=B_SPLINE_CURVE_WITH_KNOTS ( 'NONE', 3,
 ( #15803, #26518, #834, #11556, #8886, #19903 ),
 .UNSPECIFIED., .F., .F.,
 ( 4, 2, 4 ),
 ( 0.2376120521391529850, 0.2390783382518560096, 0.2405446243645580073 ),
 .UNSPECIFIED. ) ;
#22274=CIRCLE ( 'NONE', #25901, 0.5393700787401575214 ) ;
#22288=CARTESIAN_POINT ( 'NONE',  ( 0.4061284506583976994, -0.2351468520617074898, 0.1992125984251968684 ) ) ;
#22293=CARTESIAN_POINT ( 'NONE',  ( -0.4622619257814448712, 0.08092139668561793009, 0.1992125984251968684 ) ) ;
#22304=DIRECTION ( 'NONE',  ( 0.000000000000000000, 0.000000000000000000, 1.000000000000000000 ) ) ;
#22316=CARTESIAN_POINT ( 'NONE',  ( 0.0005189969344232283309, 0.3771649972486724733, 0.07637795275590551769 ) ) ;
#22317=CARTESIAN_POINT ( 'NONE',  ( -0.3073078020562972634, 0.3671449284697080873, 0.1920935997041830212 ) ) ;
#22328=EDGE_CURVE ( 'NONE', #21657, #7534, #186, .T. ) ;
#22336=ORIENTED_EDGE ( 'NONE', *, *, #355, .F. ) ;
#22373=CARTESIAN_POINT ( 'NONE',  ( 0.4149306118455894365, -0.2388850582575479942, 0.08349695147658099670 ) ) ;
#22374=DIRECTION ( 'NONE',  ( 0.7660444431189780135, 0.6427876096865393629, 0.000000000000000000 ) ) ;
#22380=LINE ( 'NONE', #16175, #18614 ) ;
#22403=CARTESIAN_POINT ( 'NONE',  ( -0.4061284506584276199, -0.2351468520616558922, 0.07637795275590551769 ) ) ;
#22405=ORIENTED_EDGE ( 'NONE', *, *, #18511, .T. ) ;
#22406=ORIENTED_EDGE ( 'NONE', *, *, #5893, .T. ) ;
#22413=EDGE_CURVE ( 'NONE', #21723, #10388, #23003, .T. ) ;
#22451=CYLINDRICAL_SURFACE ( 'NONE', #27192, 0.3771653543307086909 ) ;
#22497=CARTESIAN_POINT ( 'NONE',  ( 0.2720459371704843088, 0.3242117229735830830, 0.06102165354330708891 ) ) ;
#22502=AXIS2_PLACEMENT_3D ( 'NONE', #13520, #22145, #26799 ) ;
#22511=DIRECTION ( 'NONE',  ( 0.000000000000000000, -1.000000000000000000, 0.000000000000000000 ) ) ;
#22512=EDGE_LOOP ( 'NONE', ( #7784, #14399 ) ) ;
#22516=CARTESIAN_POINT ( 'NONE',  ( -0.2720459371704843088, 0.3242117229735834716, 0.1377952755905511861 ) ) ;
#22529=DIRECTION ( 'NONE',  ( 0.000000000000000000, 0.000000000000000000, 1.000000000000000000 ) ) ;
#22543=CARTESIAN_POINT ( 'NONE',  ( 0.000000000000000000, 0.000000000000000000, 0.1377952755905511861 ) ) ;
#22561=DIRECTION ( 'NONE',  ( 0.000000000000000000, 0.000000000000000000, 1.000000000000000000 ) ) ;
#22572=EDGE_CURVE ( 'NONE', #3499, #17056, #26742, .T. ) ;
#22582=CARTESIAN_POINT ( 'NONE',  ( 0.3169330146514671709, -0.1835719822061527007, 0.08455817587548536407 ) ) ;
#22584=ORIENTED_EDGE ( 'NONE', *, *, #16975, .T. ) ;
#22594=DIRECTION ( 'NONE',  ( 0.6427876096865399180, 0.7660444431189776804, -0.000000000000000000 ) ) ;
#22602=TOROIDAL_SURFACE ( 'NONE', #24854, 0.4232283464566928832, 0.07677165354330708902 ) ;
#22607=CARTESIAN_POINT ( 'NONE',  ( -0.2997912780622380979, -0.1736589463928937815, 0.1377952755905510751 ) ) ;
#22609=AXIS2_PLACEMENT_3D ( 'NONE', #4733, #17598, #515 ) ;
#22611=VERTEX_POINT ( 'NONE', #18022 ) ;
#22619=CARTESIAN_POINT ( 'NONE',  ( -0.3430989538740937816, 0.06100393589341226996, 0.1589462317956309712 ) ) ;
#22627=DIRECTION ( 'NONE',  ( 0.000000000000000000, 0.000000000000000000, 1.000000000000000000 ) ) ;
#22628=ORIENTED_EDGE ( 'NONE', *, *, #17874, .T. ) ;
#22631=CARTESIAN_POINT ( 'NONE',  ( 0.000000000000000000, 0.000000000000000000, 0.07637795275590551769 ) ) ;
#22644=ORIENTED_EDGE ( 'NONE', *, *, #24883, .F. ) ;
#22645=AXIS2_PLACEMENT_3D ( 'NONE', #4702, #11759, #26726 ) ;
#22710=DIRECTION ( 'NONE',  ( 0.000000000000000000, -1.000000000000000000, 0.000000000000000000 ) ) ;
#22715=CARTESIAN_POINT ( 'NONE',  ( 0.1285103288269283661, -0.3545966721392122545, 0.1992125984251968684 ) ) ;
#22717=CARTESIAN_POINT ( 'NONE',  ( -0.0005189969344232283309, 0.3771649972486724733, 0.1992125984251968684 ) ) ;
#22724=ORIENTED_EDGE ( 'NONE', *, *, #9281, .T. ) ;
#22736=VERTEX_POINT ( 'NONE', #22717 ) ;
#22739=CARTESIAN_POINT ( 'NONE',  ( -0.3020979083623086536, 0.3591256245825952265, 0.1992125984251968684 ) ) ;
#22744=TOROIDAL_SURFACE ( 'NONE', #7392, 0.3070866141732283561, 0.01181102362204724393 ) ;
#22752=ORIENTED_EDGE ( 'NONE', *, *, #25747, .F. ) ;
#22758=EDGE_CURVE ( 'NONE', #24304, #11701, #500, .T. ) ;
#22770=CARTESIAN_POINT ( 'NONE',  ( 0.000000000000000000, 0.000000000000000000, 0.1377952755905511861 ) ) ;
#22786=ORIENTED_EDGE ( 'NONE', *, *, #17363, .T. ) ;
#22788=DIRECTION ( 'NONE',  ( 0.000000000000000000, 0.000000000000000000, 1.000000000000000000 ) ) ;
#22793=CARTESIAN_POINT ( 'NONE',  ( -0.4308867145620936534, -0.2480839813580091591, 0.1140743250925834867 ) ) ;
#22800=ORIENTED_EDGE ( 'NONE', *, *, #3387, .F. ) ;
#22840=EDGE_CURVE ( 'NONE', #3499, #17056, #23637, .T. ) ;
#22850=EDGE_CURVE ( 'NONE', #10277, #12575, #24930, .T. ) ;
#22854=DIRECTION ( 'NONE',  ( 0.000000000000000000, 0.000000000000000000, 1.000000000000000000 ) ) ;
#22860=CARTESIAN_POINT ( 'NONE',  ( 0.5393700787401575214, 0.000000000000000000, 0.01181102362204724393 ) ) ;
#22874=ORIENTED_EDGE ( 'NONE', *, *, #16272, .F. ) ;
#22893=CARTESIAN_POINT ( 'NONE',  ( 0.1603262695921761627, -0.4410554214326614098, 0.1992150590373740204 ) ) ;
#22900=DIRECTION ( 'NONE',  ( 0.000000000000000000, 0.000000000000000000, 1.000000000000000000 ) ) ;
#22911=CARTESIAN_POINT ( 'NONE',  ( 0.1247869790659374006, -0.3443449117970123208, 0.1910323753032946992 ) ) ;
#22912=ADVANCED_FACE ( 'NONE', ( #17609, #13095 ), #13229, .T. ) ;
#22922=CARTESIAN_POINT ( 'NONE',  ( -0.3002886982018051487, -0.1727973894384558229, 0.1377952755905512416 ) ) ;
#22928=AXIS2_PLACEMENT_3D ( 'NONE', #24846, #24421, #5066 ) ;
#22937=DIRECTION ( 'NONE',  ( 1.000000000000000000, 0.000000000000000000, 0.000000000000000000 ) ) ;
#22942=CARTESIAN_POINT ( 'NONE',  ( -0.3665264996331779601, -0.2116141732283464416, 0.1377952755905511861 ) ) ;
#22967=ORIENTED_EDGE ( 'NONE', *, *, #26389, .F. ) ;
#22983=TOROIDAL_SURFACE ( 'NONE', #25700, 0.5393700787401575214, 0.01181102362204724393 ) ;
#22991=DIRECTION ( 'NONE',  ( 0.000000000000000000, 0.000000000000000000, -1.000000000000000000 ) ) ;
#22994=FACE_OUTER_BOUND ( 'NONE', #26734, .T. ) ;
#23003=CIRCLE ( 'NONE', #10814, 0.07677165354330708902 ) ;
#23011=ORIENTED_EDGE ( 'NONE', *, *, #8672, .T. ) ;
#23029=VERTEX_POINT ( 'NONE', #18139 ) ;
#23040=ADVANCED_FACE ( 'NONE', ( #15912, #9690 ), #18430, .T. ) ;
#23048=CARTESIAN_POINT ( 'NONE',  ( 0.000000000000000000, 0.5511811023622047445, 0.2637795275590551491 ) ) ;
#23054=CARTESIAN_POINT ( 'NONE',  ( -0.0005789221761808661720, 0.4692909815006409691, 0.1992125984251968684 ) ) ;
#23069=FACE_OUTER_BOUND ( 'NONE', #946, .T. ) ;
#23071=ORIENTED_EDGE ( 'NONE', *, *, #23983, .T. ) ;
#23075=ADVANCED_FACE ( 'NONE', ( #6192 ), #19578, .F. ) ;
#23080=ORIENTED_EDGE ( 'NONE', *, *, #25526, .F. ) ;
#23085=DIRECTION ( 'NONE',  ( 0.000000000000000000, 1.000000000000000000, 0.000000000000000000 ) ) ;
#23096=VERTEX_POINT ( 'NONE', #5753 ) ;
#23103=EDGE_CURVE ( 'NONE', #1637, #8715, #15015, .T. ) ;
#23112=CARTESIAN_POINT ( 'NONE',  ( 0.3018020646414488750, 0.3593743330771480560, 0.1992150590373740204 ) ) ;
#23117=AXIS2_PLACEMENT_3D ( 'NONE', #24557, #848, #17783 ) ;
#23122=ORIENTED_EDGE ( 'NONE', *, *, #2323, .F. ) ;
#23124=CARTESIAN_POINT ( 'NONE',  ( 0.000000000000000000, 0.000000000000000000, 0.1377952755905511861 ) ) ;
#23137=FACE_OUTER_BOUND ( 'NONE', #4357, .T. ) ;
#23143=CARTESIAN_POINT ( 'NONE',  ( -0.3012109481301850633, 0.3598698725862389813, 0.07637795275590551769 ) ) ;
#23152=CARTESIAN_POINT ( 'NONE',  ( -0.0004974201395674844595, 0.3464563358313497154, 0.1276989850599299925 ) ) ;
#23162=EDGE_CURVE ( 'NONE', #17199, #14009, #20219, .T. ) ;
#23229=DIRECTION ( 'NONE',  ( -0.1736481776669310251, -0.9848077530122080203, 0.000000000000000000 ) ) ;
#23237=CARTESIAN_POINT ( 'NONE',  ( 0.000000000000000000, 0.4692913385826771866, -3.278217716535432842E-17 ) ) ;
#23246=EDGE_CURVE ( 'NONE', #12575, #16738, #25310, .T. ) ;
#23247=AXIS2_PLACEMENT_3D ( 'NONE', #25919, #10376, #6170 ) ;
#23274=CIRCLE ( 'NONE', #687, 0.4692913385826771866 ) ;
#23282=AXIS2_PLACEMENT_3D ( 'NONE', #4266, #25453, #19231 ) ;
#23284=FACE_OUTER_BOUND ( 'NONE', #3939, .T. ) ;
#23288=EDGE_LOOP ( 'NONE', ( #14968, #5504, #24955, #3407, #11803, #18325 ) ) ;
#23299=AXIS2_PLACEMENT_3D ( 'NONE', #24559, #7338, #11852 ) ;
#23313=EDGE_LOOP ( 'NONE', ( #6061, #7815, #14402, #10122, #16054, #24980 ) ) ;
#23337=CARTESIAN_POINT ( 'NONE',  ( 0.3264619303874873313, -0.1888818218344748001, 0.07637630750536809898 ) ) ;
#23347=EDGE_CURVE ( 'NONE', #10367, #2190, #23456, .T. ) ;
#23349=ORIENTED_EDGE ( 'NONE', *, *, #19159, .T. ) ;
#23369=VERTEX_POINT ( 'NONE', #15013 ) ;
#23370=EDGE_CURVE ( 'NONE', #14826, #3213, #11902, .T. ) ;
#23382=CARTESIAN_POINT ( 'NONE',  ( -0.3432721300506699214, 0.06002180498064106640, 0.1166443193921996718 ) ) ;
#23383=DIRECTION ( 'NONE',  ( 0.000000000000000000, 0.000000000000000000, 1.000000000000000000 ) ) ;
#23387=VERTEX_POINT ( 'NONE', #9038 ) ;
#23398=CARTESIAN_POINT ( 'NONE',  ( -0.1599629598573824862, -0.4411872753631803090, 0.07637795275590551769 ) ) ;
#23405=VERTEX_POINT ( 'NONE', #10606 ) ;
#23407=VERTEX_POINT ( 'NONE', #449 ) ;
#23411=CARTESIAN_POINT ( 'NONE',  ( 0.4067073728345788064, -0.2341441294389338956, 0.1992125984251968684 ) ) ;
#23425=CIRCLE ( 'NONE', #27012, 0.07677362204724409722 ) ;
#23428=DIRECTION ( 'NONE',  ( 0.7660444431189775694, -0.6427876096865398070, 0.000000000000000000 ) ) ;
#23434=ORIENTED_EDGE ( 'NONE', *, *, #16544, .F. ) ;
#23443=CARTESIAN_POINT ( 'NONE',  ( 0.000000000000000000, 0.000000000000000000, 0.1377952755905511861 ) ) ;
#23456=CIRCLE ( 'NONE', #27041, 0.3771653543307086909 ) ;
#23460=ORIENTED_EDGE ( 'NONE', *, *, #21081, .T. ) ;
#23465=ADVANCED_FACE ( 'NONE', ( #17119, #2542 ), #11164, .T. ) ;
#23485=ORIENTED_EDGE ( 'NONE', *, *, #22135, .F. ) ;
#23486=AXIS2_PLACEMENT_3D ( 'NONE', #13132, #10743, #17242 ) ;
#23489=EDGE_CURVE ( 'NONE', #24104, #21708, #19345, .T. ) ;
#23492=CARTESIAN_POINT ( 'NONE',  ( 0.2350342994840594057, 0.2808987121547457666, 0.1910323753025394145 ) ) ;
#23510=CARTESIAN_POINT ( 'NONE',  ( 0.1196556571321023277, -0.3272932875281243104, 0.1589462317991687523 ) ) ;
#23511=CARTESIAN_POINT ( 'NONE',  ( -0.1180276236025431108, -0.3257325899126712887, 0.1478915661198716980 ) ) ;
#23535=EDGE_LOOP ( 'NONE', ( #14451, #15011 ) ) ;
#23555=DIRECTION ( 'NONE',  ( 0.000000000000000000, 0.000000000000000000, 1.000000000000000000 ) ) ;
#23560=ADVANCED_FACE ( 'NONE', ( #16107, #573 ), #24699, .T. ) ;
#23581=ADVANCED_FACE ( 'NONE', ( #10288, #6080 ), #1825, .T. ) ;
#23588=ORIENTED_EDGE ( 'NONE', *, *, #24698, .T. ) ;
#23593=CARTESIAN_POINT ( 'NONE',  ( 0.4714076450716228051, 0.08371568475168257584, 0.1920935997044048160 ) ) ;
#23597=TOROIDAL_SURFACE ( 'NONE', #5525, 0.4232283464566928832, 0.07677165354330708902 ) ;
#23598=CARTESIAN_POINT ( 'NONE',  ( 0.000000000000000000, 0.000000000000000000, 0.1377952755905511861 ) ) ;
#23614=CARTESIAN_POINT ( 'NONE',  ( -0.4067073728345488304, -0.2341441294389850492, 0.07637795275590551769 ) ) ;
#23616=ORIENTED_EDGE ( 'NONE', *, *, #21914, .T. ) ;
#23623=DIRECTION ( 'NONE',  ( 1.000000000000000000, 0.000000000000000000, 0.000000000000000000 ) ) ;
#23628=CARTESIAN_POINT ( 'NONE',  ( 0.000000000000000000, 0.4232283464566928832, -3.341531889763779686E-17 ) ) ;
#23637=CIRCLE ( 'NONE', #25884, 0.07677362204724409722 ) ;
#23672=ORIENTED_EDGE ( 'NONE', *, *, #1409, .T. ) ;
#23673=TOROIDAL_SURFACE ( 'NONE', #4686, 0.5393700787401575214, 0.01181102362204724393 ) ;
#23681=CARTESIAN_POINT ( 'NONE',  ( 0.1447526197146039584, -0.3977045540727763839, 0.1377952755905511861 ) ) ;
#23701=CARTESIAN_POINT ( 'NONE',  ( 0.3529960615039756111, 0.06172929298871281112, 0.09506557083684616383 ) ) ;
#23712=CARTESIAN_POINT ( 'NONE',  ( -0.2720459371704843088, 0.3242117229735834716, 0.1377952755905511861 ) ) ;
#23717=ORIENTED_EDGE ( 'NONE', *, *, #6964, .F. ) ;
#23755=CARTESIAN_POINT ( 'NONE',  ( 0.000000000000000000, 0.000000000000000000, -3.278217716535432842E-17 ) ) ;
#23757=FACE_OUTER_BOUND ( 'NONE', #3779, .T. ) ;
#23764=EDGE_CURVE ( 'NONE', #2394, #19464, #9508, .T. ) ;
#23776=ORIENTED_EDGE ( 'NONE', *, *, #16746, .T. ) ;
#23781=CARTESIAN_POINT ( 'NONE',  ( 0.1257482708760437329, -0.3439950301959718848, 0.1910323753063126184 ) ) ;
#23790=AXIS2_PLACEMENT_3D ( 'NONE', #16927, #1799, #24712 ) ;
#23808=CARTESIAN_POINT ( 'NONE',  ( -0.3020979083623086536, 0.3591256245825952265, 0.1992125984251968684 ) ) ;
#23816=ORIENTED_EDGE ( 'NONE', *, *, #16418, .F. ) ;
#23818=B_SPLINE_CURVE_WITH_KNOTS ( 'NONE', 3,
 ( #11158, #27608, #10354, #17649, #13280, #10491, #26036, #8393, #15425, #17141 ),
 .UNSPECIFIED., .F., .F.,
 ( 4, 2, 2, 2, 4 ),
 ( 0.000000000000000000, 0.2500000000000001665, 0.5000000000000003331, 0.7500000000000001110, 1.000000000000000000 ),
 .UNSPECIFIED. ) ;
#23831=B_SPLINE_CURVE_WITH_KNOTS ( 'NONE', 3,
 ( #25050, #12755, #27316, #18968, #1457, #7826 ),
 .UNSPECIFIED., .F., .F.,
 ( 4, 2, 4 ),
 ( 0.5000000000000000000, 0.7500000000000000000, 1.000000000000000000 ),
 .UNSPECIFIED. ) ;
#23832=ORIENTED_EDGE ( 'NONE', *, *, #6126, .F. ) ;
#23848=CARTESIAN_POINT ( 'NONE',  ( 0.3665264996331779601, -0.2116141732283464416, 0.1377952755905511861 ) ) ;
#23856=AXIS2_PLACEMENT_3D ( 'NONE', #22770, #3842, #3395 ) ;
#23890=CARTESIAN_POINT ( 'NONE',  ( 0.3411065095061437402, 0.06065137456822567580, 0.1478915661283759231 ) ) ;
#23899=CARTESIAN_POINT ( 'NONE',  ( -0.0005114926878551800428, 0.3662580330867932221, 0.1910323753037873884 ) ) ;
#23900=CARTESIAN_POINT ( 'NONE',  ( 0.4792984784118546893, 0.08391448672373898188, 0.1827409795125537750 ) ) ;
#23902=CARTESIAN_POINT ( 'NONE',  ( -0.4066108233583488052, -0.2343118354750405585, 0.1992142434433716580 ) ) ;
#23905=CARTESIAN_POINT ( 'NONE',  ( -0.5393700787401575214, 6.677700066216866815E-17, -3.278217716535432842E-17 ) ) ;
#23911=EDGE_CURVE ( 'NONE', #13649, #6594, #20022, .T. ) ;
#23918=CARTESIAN_POINT ( 'NONE',  ( 0.1189624676717044027, -0.3253923344978161825, 0.1478915661284414818 ) ) ;
#23922=( LENGTH_UNIT ( ) NAMED_UNIT ( * ) SI_UNIT ( $, .METRE. ) ) ;
#23942=B_SPLINE_CURVE_WITH_KNOTS ( 'NONE', 3,
 ( #26008, #23899, #4536, #6380, #9037, #18040 ),
 .UNSPECIFIED., .F., .F.,
 ( 4, 2, 4 ),
 ( 0.000000000000000000, 0.2500000000000000000, 0.5000000000000000000 ),
 .UNSPECIFIED. ) ;
#23945=ORIENTED_EDGE ( 'NONE', *, *, #23993, .F. ) ;
#23968=ORIENTED_EDGE ( 'NONE', *, *, #20798, .T. ) ;
#23978=ORIENTED_EDGE ( 'NONE', *, *, #8643, .T. ) ;
#23983=EDGE_CURVE ( 'NONE', #8124, #26656, #2753, .T. ) ;
#23993=EDGE_CURVE ( 'NONE', #4856, #2522, #12235, .T. ) ;
#23997=DIRECTION ( 'NONE',  ( 1.224646799147353207E-16, 1.000000000000000000, -0.000000000000000000 ) ) ;
#24013=EDGE_CURVE ( 'NONE', #13133, #17199, #7176, .T. ) ;
#24023=CARTESIAN_POINT ( 'NONE',  ( 0.4792984784026986245, 0.08391448672215147397, 0.09284957165657019285 ) ) ;
#24052=AXIS2_PLACEMENT_3D ( 'NONE', #19637, #6916, #308 ) ;
#24053=VERTEX_POINT ( 'NONE', #1273 ) ;
#24059=TOROIDAL_SURFACE ( 'NONE', #15927, 0.4232283464566928832, 0.07677165354330708902 ) ;
#24065=ORIENTED_EDGE ( 'NONE', *, *, #5625, .T. ) ;
#24067=CYLINDRICAL_SURFACE ( 'NONE', #22645, 0.5511811023622047445 ) ;
#24071=CARTESIAN_POINT ( 'NONE',  ( 0.3665264996331779601, -0.2116141732283464416, 0.1377952755905511861 ) ) ;
#24079=EDGE_CURVE ( 'NONE', #9569, #3368, #1137, .T. ) ;
#24091=ORIENTED_EDGE ( 'NONE', *, *, #24698, .F. ) ;
#24101=CARTESIAN_POINT ( 'NONE',  ( 0.000000000000000000, 0.000000000000000000, 0.2374015748031496065 ) ) ;
#24103=ORIENTED_EDGE ( 'NONE', *, *, #12206, .T. ) ;
#24104=VERTEX_POINT ( 'NONE', #11719 ) ;
#24131=CARTESIAN_POINT ( 'NONE',  ( -0.3070866141732283561, 3.760726391082423050E-17, 0.2637795275590551491 ) ) ;
#24133=B_SPLINE_CURVE_WITH_KNOTS ( 'NONE', 3,
 ( #24597, #27160, #16410, #12166, #18073, #1171 ),
 .UNSPECIFIED., .F., .F.,
 ( 4, 2, 4 ),
 ( 0.6902184472752670441, 0.6915327610580710438, 0.6928470748408740443 ),
 .UNSPECIFIED. ) ;
#24138=CARTESIAN_POINT ( 'NONE',  ( 0.000000000000000000, 0.000000000000000000, 0.1992125984251968684 ) ) ;
#24142=B_SPLINE_CURVE_WITH_KNOTS ( 'NONE', 3,
 ( #6169, #10801, #2042, #14795, #19418, #23398 ),
 .UNSPECIFIED., .F., .F.,
 ( 4, 2, 4 ),
 ( 0.2376120521391529850, 0.2390783382518560096, 0.2405446243645580073 ),
 .UNSPECIFIED. ) ;
#24143=( NAMED_UNIT ( * ) SI_UNIT ( $, .STERADIAN. ) SOLID_ANGLE_UNIT ( ) ) ;
#24162=CARTESIAN_POINT ( 'NONE',  ( -0.4063220079890716430, -0.2348123150948748239, 0.1992150590373740204 ) ) ;
#24164=CARTESIAN_POINT ( 'NONE',  ( -0.3218517393628410050, 0.3826375019110230258, 0.1496602734613065311 ) ) ;
#24171=CIRCLE ( 'NONE', #21480, 0.07677362204724408334 ) ;
#24175=ADVANCED_FACE ( 'NONE', ( #12138, #18770 ), #20763, .T. ) ;
#24187=SURFACE_STYLE_FILL_AREA ( #26295 ) ;
#24192=ORIENTED_EDGE ( 'NONE', *, *, #19595, .F. ) ;
#24198=DIRECTION ( 'NONE',  ( 1.000000000000000000, 0.000000000000000000, 0.000000000000000000 ) ) ;
#24200=DIRECTION ( 'NONE',  ( 1.000000000000000000, 0.000000000000000000, 0.000000000000000000 ) ) ;
#24203=TOROIDAL_SURFACE ( 'NONE', #19713, 0.4232283464566928832, 0.07677165354330708902 ) ;
#24211=DIRECTION ( 'NONE',  ( 0.000000000000000000, 0.000000000000000000, 1.000000000000000000 ) ) ;
#24217=CARTESIAN_POINT ( 'NONE',  ( 0.4232283464566928832, 0.000000000000000000, 0.1377952755905511861 ) ) ;
#24223=CARTESIAN_POINT ( 'NONE',  ( 0.000000000000000000, 0.000000000000000000, 0.07637795275590551769 ) ) ;
#24265=CIRCLE ( 'NONE', #6244, 0.2952755905511810774 ) ;
#24268=CARTESIAN_POINT ( 'NONE',  ( 0.4327133464951135045, -0.2505177833314600200, 0.1496602734566857273 ) ) ;
#24269=ORIENTED_EDGE ( 'NONE', *, *, #12206, .F. ) ;
#24287=DIRECTION ( 'NONE',  ( 0.000000000000000000, 1.000000000000000000, 0.000000000000000000 ) ) ;
#24304=VERTEX_POINT ( 'NONE', #7722 ) ;
#24316=CARTESIAN_POINT ( 'NONE',  ( -0.3265485372158890010, -0.1887320510662011952, 0.1992150590373740204 ) ) ;
#24328=EDGE_CURVE ( 'NONE', #8023, #26363, #3305, .T. ) ;
#24329=CARTESIAN_POINT ( 'NONE',  ( 0.000000000000000000, 0.000000000000000000, 0.07637795275590551769 ) ) ;
#24331=CARTESIAN_POINT ( 'NONE',  ( 0.3020979083623086536, 0.3591256245825952265, 0.1992125984251968684 ) ) ;
#24379=ORIENTED_EDGE ( 'NONE', *, *, #20207, .T. ) ;
#24419=CARTESIAN_POINT ( 'NONE',  ( 0.3464566929133857665, 0.000000000000000000, 0.1377952755905511584 ) ) ;
#24421=DIRECTION ( 'NONE',  ( 0.000000000000000000, 0.000000000000000000, 1.000000000000000000 ) ) ;
#24441=AXIS2_PLACEMENT_3D ( 'NONE', #8836, #12526, #25377 ) ;
#24455=CARTESIAN_POINT ( 'NONE',  ( 0.1247869790670923795, -0.3443449118002068210, 0.08455817587526011370 ) ) ;
#24463=EDGE_CURVE ( 'NONE', #10706, #14762, #18222, .T. ) ;
#24468=CARTESIAN_POINT ( 'NONE',  ( -0.1189624676717059848, -0.3253923344978159604, 0.1377952755905513249 ) ) ;
#24471=AXIS2_PLACEMENT_3D ( 'NONE', #6956, #1559, #18781 ) ;
#24491=B_SPLINE_CURVE_WITH_KNOTS ( 'NONE', 3,
 ( #27415, #19351, #7924, #8350, #6098, #1975 ),
 .UNSPECIFIED., .F., .F.,
 ( 4, 2, 4 ),
 ( 0.2291966065698869959, 0.2305109203526909956, 0.2318252341354939960 ),
 .UNSPECIFIED. ) ;
#24504=AXIS2_PLACEMENT_3D ( 'NONE', #13989, #22594, #16248 ) ;
#24508=EDGE_CURVE ( 'NONE', #11010, #24104, #16586, .T. ) ;
#24518=EDGE_LOOP ( 'NONE', ( #21645, #6760, #4716, #7713, #8699, #19669 ) ) ;
#24546=CARTESIAN_POINT ( 'NONE',  ( 0.2720459371704843088, 0.3242117229735830830, 0.2145688976377952695 ) ) ;
#24549=ORIENTED_EDGE ( 'NONE', *, *, #24328, .T. ) ;
#24557=CARTESIAN_POINT ( 'NONE',  ( 0.000000000000000000, 0.000000000000000000, 0.1992125984251968684 ) ) ;
#24558=CARTESIAN_POINT ( 'NONE',  ( -0.4621283342336243716, 0.08168108835551378399, 0.1992150590373740204 ) ) ;
#24559=CARTESIAN_POINT ( 'NONE',  ( 0.000000000000000000, 0.000000000000000000, 0.1992125984251968684 ) ) ;
#24571=CARTESIAN_POINT ( 'NONE',  ( 0.1608692170994283632, -0.4408576787418519993, 0.1992142434433712694 ) ) ;
#24573=CARTESIAN_POINT ( 'NONE',  ( -5.645730259564185549E-17, 0.4692913385826772976, 0.07637549214372836570 ) ) ;
#24578=EDGE_CURVE ( 'NONE', #8859, #13133, #12387, .T. ) ;
#24586=ORIENTED_EDGE ( 'NONE', *, *, #19573, .F. ) ;
#24596=AXIS2_PLACEMENT_3D ( 'NONE', #24138, #17765, #19898 ) ;
#24597=CARTESIAN_POINT ( 'NONE',  ( -0.1294857240059045234, -0.3542416573274181357, 0.1992125984251968684 ) ) ;
#24607=ADVANCED_FACE ( 'NONE', ( #20370, #15998 ), #14168, .T. ) ;
#24623=CARTESIAN_POINT ( 'NONE',  ( -0.2223167940359792594, 0.2657206863494902538, 0.1377952755905513249 ) ) ;
#24639=VERTEX_POINT ( 'NONE', #11036 ) ;
#24660=ADVANCED_FACE ( 'NONE', ( #12290 ), #12059, .F. ) ;
#24666=ADVANCED_FACE ( 'NONE', ( #21695, #17311 ), #27779, .T. ) ;
#24671=CARTESIAN_POINT ( 'NONE',  ( -6.750021727583836750E-17, -0.5511811023622047445, 0.2637795275590551491 ) ) ;
#24673=CARTESIAN_POINT ( 'NONE',  ( -0.1447526197146041249, -0.3977045540727763839, 0.1377952755905511861 ) ) ;
#24691=CARTESIAN_POINT ( 'NONE',  ( 0.1189624676717049440, -0.3253923344978161825, 0.1377952755905510474 ) ) ;
#24698=EDGE_CURVE ( 'NONE', #17997, #1348, #3047, .T. ) ;
#24699=SPHERICAL_SURFACE ( 'NONE', #24504, 0.07677362204724409722 ) ;
#24702=ORIENTED_EDGE ( 'NONE', *, *, #24578, .T. ) ;
#24708=CARTESIAN_POINT ( 'NONE',  ( -0.2223167940359789541, 0.2657206863494903093, 0.1276989850623086176 ) ) ;
#24712=DIRECTION ( 'NONE',  ( 1.000000000000000000, 0.000000000000000000, 0.000000000000000000 ) ) ;
#24715=B_SPLINE_CURVE_WITH_KNOTS ( 'NONE', 3,
 ( #19341, #21334, #27555, #8196, #25424, #14726 ),
 .UNSPECIFIED., .F., .F.,
 ( 4, 2, 4 ),
 ( 0.2376120521391529850, 0.2390783382518550104, 0.2405446243645580073 ),
 .UNSPECIFIED. ) ;
#24719=B_SPLINE_CURVE_WITH_KNOTS ( 'NONE', 3,
 ( #23143, #10544, #12539, #21154, #1798, #19025 ),
 .UNSPECIFIED., .F., .F.,
 ( 4, 2, 4 ),
 ( 0.2376120521390029938, 0.2390783382518560096, 0.2405446243647090254 ),
 .UNSPECIFIED. ) ;
#24724=CARTESIAN_POINT ( 'NONE',  ( -0.3411065095061439068, 0.06065137456822528722, 0.1478915661262500403 ) ) ;
#24730=VECTOR ( 'NONE', #25486, 39.37007874015748143 ) ;
#24731=FACE_OUTER_BOUND ( 'NONE', #108, .T. ) ;
#24740=CARTESIAN_POINT ( 'NONE',  ( -0.3713448905834433322, 0.06600512665679449109, 0.07637795275590551769 ) ) ;
#24753=CARTESIAN_POINT ( 'NONE',  ( 0.000000000000000000, 0.000000000000000000, 0.1992125984251968684 ) ) ;
#24777=EDGE_CURVE ( 'NONE', #23387, #12348, #7478, .T. ) ;
#24781=B_SPLINE_CURVE_WITH_KNOTS ( 'NONE', 3,
 ( #25876, #4404, #19512, #6666 ),
 .UNSPECIFIED., .F., .F.,
 ( 4, 4 ),
 ( 0.7157687286427140139, 0.7172350147555668354 ),
 .UNSPECIFIED. ) ;
#24790=CIRCLE ( 'NONE', #27065, 0.3771653543307086909 ) ;
#24815=VERTEX_POINT ( 'NONE', #21179 ) ;
#24831=CARTESIAN_POINT ( 'NONE',  ( 0.3100894960467185379, -0.1796141127317343322, 0.09506557083533939689 ) ) ;
#24845=DIRECTION ( 'NONE',  ( 0.000000000000000000, 1.000000000000000000, 0.000000000000000000 ) ) ;
#24846=CARTESIAN_POINT ( 'NONE',  ( 0.000000000000000000, 0.000000000000000000, 0.1377952755905511861 ) ) ;
#24848=CARTESIAN_POINT ( 'NONE',  ( 0.000000000000000000, 0.000000000000000000, 0.07637795275590551769 ) ) ;
#24853=CARTESIAN_POINT ( 'NONE',  ( 0.4062254136079394562, -0.2349793847444826833, 0.07637630773773071424 ) ) ;
#24854=AXIS2_PLACEMENT_3D ( 'NONE', #26745, #18100, #9222 ) ;
#24864=DIRECTION ( 'NONE',  ( 0.000000000000000000, 1.000000000000000000, 0.000000000000000000 ) ) ;
#24867=EDGE_LOOP ( 'NONE', ( #24192, #18315, #1524, #18467 ) ) ;
#24872=CARTESIAN_POINT ( 'NONE',  ( -0.3002886982018051487, -0.1727973894384558229, 0.1377952755905512416 ) ) ;
#24883=EDGE_CURVE ( 'NONE', #21302, #16931, #13274, .T. ) ;
#24886=CARTESIAN_POINT ( 'NONE',  ( 0.000000000000000000, 0.000000000000000000, 0.2637795275590551491 ) ) ;
#24902=CARTESIAN_POINT ( 'NONE',  ( 0.3070866141732283561, 0.000000000000000000, 0.2637795275590551491 ) ) ;
#24904=CARTESIAN_POINT ( 'NONE',  ( -0.4308867145613631822, -0.2480839813575886066, 0.1615162260909178693 ) ) ;
#24907=CARTESIAN_POINT ( 'NONE',  ( 0.3713448905834433322, 0.06600512665679410251, 0.07637795275590551769 ) ) ;
#24910=CARTESIAN_POINT ( 'NONE',  ( 0.1285103288269283661, -0.3545966721392122545, 0.07637795275590551769 ) ) ;
#24925=CARTESIAN_POINT ( 'NONE',  ( 0.3412792617076849666, 0.05967164814832574826, 0.1478915661242290458 ) ) ;
#24930=CIRCLE ( 'NONE', #10968, 0.5511811023622047445 ) ;
#24941=DIRECTION ( 'NONE',  ( -0.4999999999999995004, -0.8660254037844390407, 0.000000000000000000 ) ) ;
#24955=ORIENTED_EDGE ( 'NONE', *, *, #9281, .F. ) ;
#24960=CARTESIAN_POINT ( 'NONE',  ( -0.3268939675028499914, -0.1881330340946393564, 0.07637795275590551769 ) ) ;
#24971=CARTESIAN_POINT ( 'NONE',  ( -0.1447526197146041249, -0.3977045540727763839, 0.1377952755905511861 ) ) ;
#24980=ORIENTED_EDGE ( 'NONE', *, *, #21633, .F. ) ;
#24985=CARTESIAN_POINT ( 'NONE',  ( 0.4622619257814448712, 0.08092139668561752763, 0.1992125984251968684 ) ) ;
#24994=CARTESIAN_POINT ( 'NONE',  ( 0.1606879121749082706, -0.4409237942971039881, 0.1992150590373740204 ) ) ;
#25012=CARTESIAN_POINT ( 'NONE',  ( 0.000000000000000000, 0.000000000000000000, 0.1377952755905511861 ) ) ;
#25020=ORIENTED_EDGE ( 'NONE', *, *, #1983, .T. ) ;
#25026=CARTESIAN_POINT ( 'NONE',  ( -0.1447526197146041249, -0.3977045540727763839, 0.1377952755905511861 ) ) ;
#25028=CARTESIAN_POINT ( 'NONE',  ( -0.3002886982018052042, -0.1727973894384558229, 0.1478915661221150424 ) ) ;
#25029=EDGE_CURVE ( 'NONE', #17458, #5345, #9670, .T. ) ;
#25030=CARTESIAN_POINT ( 'NONE',  ( -0.1189624676717059848, -0.3253923344978159604, 0.1377952755905513249 ) ) ;
#25031=ORIENTED_EDGE ( 'NONE', *, *, #21603, .T. ) ;
#25032=DIRECTION ( 'NONE',  ( 0.000000000000000000, 0.000000000000000000, 1.000000000000000000 ) ) ;
#25033=EDGE_CURVE ( 'NONE', #3709, #26883, #266, .T. ) ;
#25040=VERTEX_POINT ( 'NONE', #1238 ) ;
#25050=CARTESIAN_POINT ( 'NONE',  ( 0.2223167940359795647, 0.2657206863494897542, 0.1377952755905510474 ) ) ;
#25063=AXIS2_PLACEMENT_3D ( 'NONE', #2864, #20258, #11503 ) ;
#25066=ORIENTED_EDGE ( 'NONE', *, *, #21474, .T. ) ;
#25074=ORIENTED_EDGE ( 'NONE', *, *, #25029, .T. ) ;
#25076=CARTESIAN_POINT ( 'NONE',  ( 0.3015072509068625894, 0.3596217111731054850, 0.1992150590373740204 ) ) ;
#25083=CIRCLE ( 'NONE', #11546, 0.07677362204724411110 ) ;
#25085=ORIENTED_EDGE ( 'NONE', *, *, #13100, .F. ) ;
#25104=FACE_OUTER_BOUND ( 'NONE', #1554, .T. ) ;
#25111=CIRCLE ( 'NONE', #8874, 0.2952755905511810774 ) ;
#25122=ORIENTED_EDGE ( 'NONE', *, *, #4204, .F. ) ;
#25128=CARTESIAN_POINT ( 'NONE',  ( -0.4621951630817708878, 0.08130208312399901660, 0.1992150590373740204 ) ) ;
#25130=ORIENTED_EDGE ( 'NONE', *, *, #8672, .F. ) ;
#25152=DIRECTION ( 'NONE',  ( 0.000000000000000000, 0.000000000000000000, 1.000000000000000000 ) ) ;
#25155=CARTESIAN_POINT ( 'NONE',  ( 0.1180276236025432773, -0.3257325899126712887, 0.1478915661236427093 ) ) ;
#25158=CARTESIAN_POINT ( 'NONE',  ( 0.000000000000000000, 0.000000000000000000, -3.278217716535432842E-17 ) ) ;
#25178=CARTESIAN_POINT ( 'NONE',  ( -0.1180276236025431524, -0.3257325899126714552, 0.1377952755905512139 ) ) ;
#25180=EDGE_LOOP ( 'NONE', ( #16875, #27313, #26472, #23945 ) ) ;
#25185=CARTESIAN_POINT ( 'NONE',  ( 0.3020416211901519321, -0.1738080303474756061, 0.1166443193831429581 ) ) ;
#25226=ORIENTED_EDGE ( 'NONE', *, *, #13100, .T. ) ;
#25229=DIRECTION ( 'NONE',  ( 0.9848077530122082424, 0.1736481776669299149, -0.000000000000000000 ) ) ;
#25231=EDGE_CURVE ( 'NONE', #9015, #8846, #6154, .T. ) ;
#25232=FACE_OUTER_BOUND ( 'NONE', #9617, .T. ) ;
#25242=DIRECTION ( 'NONE',  ( 0.6427876096865399180, 0.7660444431189776804, -0.000000000000000000 ) ) ;
#25247=CARTESIAN_POINT ( 'NONE',  ( -0.3267210193396165585, -0.1884333032645074957, 0.07637549214372854611 ) ) ;
#25257=CARTESIAN_POINT ( 'NONE',  ( -0.0005114926878479780130, 0.3662580330841598841, 0.08455817587928993184 ) ) ;
#25268=AXIS2_PLACEMENT_3D ( 'NONE', #20614, #5505, #20187 ) ;
#25291=EDGE_CURVE ( 'NONE', #24104, #8578, #19636, .T. ) ;
#25297=DIRECTION ( 'NONE',  ( 0.000000000000000000, -1.000000000000000000, 0.000000000000000000 ) ) ;
#25309=ORIENTED_EDGE ( 'NONE', *, *, #18871, .F. ) ;
#25310=CIRCLE ( 'NONE', #20851, 0.01181102362204724046 ) ;
#25315=CARTESIAN_POINT ( 'NONE',  ( -0.1196556571311373357, -0.3272932875254820906, 0.1589462317892271492 ) ) ;
#25317=CARTESIAN_POINT ( 'NONE',  ( 0.4622619257814448712, 0.08092139668561752763, 0.1992125984251968684 ) ) ;
#25335=DIRECTION ( 'NONE',  ( 0.7660444431189780135, 0.6427876096865393629, 0.000000000000000000 ) ) ;
#25336=ORIENTED_EDGE ( 'NONE', *, *, #18871, .T. ) ;
#25343=EDGE_CURVE ( 'NONE', #20180, #23029, #9110, .T. ) ;
#25360=ORIENTED_EDGE ( 'NONE', *, *, #25343, .T. ) ;
#25365=CARTESIAN_POINT ( 'NONE',  ( 0.0001924259990619888469, 0.4692913385826771866, 0.1992150590373740204 ) ) ;
#25373=LINE ( 'NONE', #16346, #9852 ) ;
#25377=DIRECTION ( 'NONE',  ( 0.000000000000000000, 1.000000000000000000, 0.000000000000000000 ) ) ;
#25387=CARTESIAN_POINT ( 'NONE',  ( 0.3715251363271980245, 0.06498290224717499786, 0.07637795275590551769 ) ) ;
#25402=ORIENTED_EDGE ( 'NONE', *, *, #1535, .F. ) ;
#25406=ORIENTED_EDGE ( 'NONE', *, *, #1535, .T. ) ;
#25408=EDGE_CURVE ( 'NONE', #19933, #23405, #11058, .T. ) ;
#25424=CARTESIAN_POINT ( 'NONE',  ( -0.4622285577935897893, 0.08111201067594607517, 0.07637630773773071424 ) ) ;
#25429=AXIS2_PLACEMENT_3D ( 'NONE', #1255, #5780, #20602 ) ;
#25448=ORIENTED_EDGE ( 'NONE', *, *, #22135, .T. ) ;
#25450=EDGE_LOOP ( 'NONE', ( #5298, #25938 ) ) ;
#25453=DIRECTION ( 'NONE',  ( 0.9848077530122081313, 0.1736481776669301369, -0.000000000000000000 ) ) ;
#25458=DIRECTION ( 'NONE',  ( 0.000000000000000000, -1.000000000000000000, 0.000000000000000000 ) ) ;
#25485=EDGE_LOOP ( 'NONE', ( #11549, #17461, #15890, #26611 ) ) ;
#25486=DIRECTION ( 'NONE',  ( 0.000000000000000000, 0.000000000000000000, 1.000000000000000000 ) ) ;
#25496=ORIENTED_EDGE ( 'NONE', *, *, #17482, .F. ) ;
#25497=ORIENTED_EDGE ( 'NONE', *, *, #6158, .T. ) ;
#25511=CARTESIAN_POINT ( 'NONE',  ( 0.0005789221761808661720, 0.4692909815006409691, 0.1992125984251968684 ) ) ;
#25519=CARTESIAN_POINT ( 'NONE',  ( -0.2997912780622380979, -0.1736589463928937815, 0.1377952755905510751 ) ) ;
#25522=CARTESIAN_POINT ( 'NONE',  ( 0.0005847768872433690111, 0.4787829797941601240, 0.1920935997050574051 ) ) ;
#25526=EDGE_CURVE ( 'NONE', #24815, #23096, #6564, .T. ) ;
#25547=ORIENTED_EDGE ( 'NONE', *, *, #7278, .T. ) ;
#25551=CARTESIAN_POINT ( 'NONE',  ( -0.3713448905834433322, 0.06600512665679449109, 0.1992125984251968684 ) ) ;
#25575=ORIENTED_EDGE ( 'NONE', *, *, #15081, .F. ) ;
#25576=CARTESIAN_POINT ( 'NONE',  ( 0.3263749705684267921, -0.1890319631540330891, 0.07637795275590551769 ) ) ;
#25594=CARTESIAN_POINT ( 'NONE',  ( 0.2420394123212937232, 0.2892587550802425134, 0.1992125984251968684 ) ) ;
#25601=EDGE_LOOP ( 'NONE', ( #25547, #15390, #552, #15947 ) ) ;
#25605=B_SPLINE_CURVE_WITH_KNOTS ( 'NONE', 3,
 ( #24623, #14051, #20680, #7695, #1333, #1201 ),
 .UNSPECIFIED., .F., .F.,
 ( 4, 2, 4 ),
 ( 0.5000000000000000000, 0.7500000000000000000, 1.000000000000000000 ),
 .UNSPECIFIED. ) ;
#25615=EDGE_CURVE ( 'NONE', #2190, #10904, #19239, .T. ) ;
#25626=CARTESIAN_POINT ( 'NONE',  ( -0.4211031283192478991, -0.2438048970112350611, 0.09284957166442699139 ) ) ;
#25629=CARTESIAN_POINT ( 'NONE',  ( -0.3132247436411769170, 0.3723693495138340470, 0.09284957166379273485 ) ) ;
#25644=CARTESIAN_POINT ( 'NONE',  ( -0.3015072509068622009, 0.3596217111731054850, 0.1992150590373740204 ) ) ;
#25660=CARTESIAN_POINT ( 'NONE',  ( 0.3100894960451806570, -0.1796141127308419627, 0.1805249803430634403 ) ) ;
#25669=VERTEX_POINT ( 'NONE', #6663 ) ;
#25693=CARTESIAN_POINT ( 'NONE',  ( -0.1715719712211479508, -0.4696414150086907768, 0.1496602734581923833 ) ) ;
#25696=CARTESIAN_POINT ( 'NONE',  ( -0.4622619257814448712, 0.08092139668561793009, 0.1992125984251968684 ) ) ;
#25700=AXIS2_PLACEMENT_3D ( 'NONE', #5768, #14537, #14389 ) ;
#25712=EDGE_CURVE ( 'NONE', #2591, #24815, #13463, .T. ) ;
#25719=EDGE_CURVE ( 'NONE', #8867, #20727, #17809, .T. ) ;
#25722=VERTEX_POINT ( 'NONE', #10605 ) ;
#25723=CARTESIAN_POINT ( 'NONE',  ( 0.3713448905834433322, 0.06600512665679410251, 0.1992125984251968684 ) ) ;
#25729=FACE_OUTER_BOUND ( 'NONE', #1910, .T. ) ;
#25732=CARTESIAN_POINT ( 'NONE',  ( 0.1447526197146039584, -0.3977045540727763839, 0.1377952755905511861 ) ) ;
#25740=B_SPLINE_CURVE_WITH_KNOTS ( 'NONE', 3,
 ( #6700, #4442, #11201, #484, #10646, #13052, #12908, #103, #21534, #17155 ),
 .UNSPECIFIED., .F., .F.,
 ( 4, 2, 2, 2, 4 ),
 ( 0.000000000000000000, 0.2500000000000000000, 0.5000000000000000000, 0.7500000000000000000, 1.000000000000000000 ),
 .UNSPECIFIED. ) ;
#25741=FACE_BOUND ( 'NONE', #21614, .T. ) ;
#25747=EDGE_CURVE ( 'NONE', #22736, #17040, #23942, .T. ) ;
#25756=CARTESIAN_POINT ( 'NONE',  ( -0.2428345617565149384, 0.2885915454824177218, 0.1992125984251968684 ) ) ;
#25772=VECTOR ( 'NONE', #9503, 39.37007874015748143 ) ;
#25779=ORIENTED_EDGE ( 'NONE', *, *, #25615, .F. ) ;
#25781=CIRCLE ( 'NONE', #23486, 0.3771653543307086909 ) ;
#25796=CARTESIAN_POINT ( 'NONE',  ( 0.2997912780622380424, -0.1736589463928938648, 0.1478915661253835667 ) ) ;
#25800=CARTESIAN_POINT ( 'NONE',  ( 0.0005980912172697295821, 0.4999996422873388968, 0.1259302777261152306 ) ) ;
#25802=FACE_BOUND ( 'NONE', #15764, .T. ) ;
#25814=AXIS2_PLACEMENT_3D ( 'NONE', #21631, #19501, #26003 ) ;
#25832=CARTESIAN_POINT ( 'NONE',  ( -0.3412792617076848001, 0.05967164814832656705, 0.1478915661216427813 ) ) ;
#25866=FACE_OUTER_BOUND ( 'NONE', #12091, .T. ) ;
#25872=CARTESIAN_POINT ( 'NONE',  ( 0.4716107359567087154, 0.08256389912760109251, 0.1920935997017693131 ) ) ;
#25875=CLOSED_SHELL ( 'NONE', ( #17756, #3469, #13438, #13741, #9777, #17415, #18943, #7854, #23075, #8987, #1318, #15344, #10397, #16962, #12695, #230, #2617, #2539, #22912, #19400, #13272, #4342, #5365, #8022, #18412, #5723, #21925, #12447, #16464, #8994, #2445, #13378, #9616, #13171, #17600, #24175, #4305, #24660, #14166, #5110, #18148, #17322, #16493, #19381, #21241, #19430, #18978, #18962, #6774, #3900, #26420, #18267, #10432, #21832, #27437, #7428, #24666, #24607, #4419, #23040, #26092, #23560, #8950, #14435, #509, #635, #4230, #23465, #2666, #23581, #20408, #14900 ) ) ;
#25876=CARTESIAN_POINT ( 'NONE',  ( -0.0005789221761808661720, 0.4692909815006409691, 0.1992125984251968684 ) ) ;
#25884=AXIS2_PLACEMENT_3D ( 'NONE', #23712, #11384, #6609 ) ;
#25896=CARTESIAN_POINT ( 'NONE',  ( -0.3715251363271980245, 0.06498290224717540031, 0.1992125984251968684 ) ) ;
#25901=AXIS2_PLACEMENT_3D ( 'NONE', #6257, #10336, #8093 ) ;
#25915=DIRECTION ( 'NONE',  ( 0.000000000000000000, 1.000000000000000000, 0.000000000000000000 ) ) ;
#25919=CARTESIAN_POINT ( 'NONE',  ( 0.000000000000000000, 0.000000000000000000, 0.01181102362204724393 ) ) ;
#25921=CARTESIAN_POINT ( 'NONE',  ( -0.3012109481301850633, 0.3598698725862389813, 0.1992125984251968684 ) ) ;
#25922=CARTESIAN_POINT ( 'NONE',  ( -0.0001724821237274612798, 0.3771653543307086909, 0.1992150590373740204 ) ) ;
#25929=CARTESIAN_POINT ( 'NONE',  ( 0.000000000000000000, 0.000000000000000000, 0.07637795275590551769 ) ) ;
#25933=CARTESIAN_POINT ( 'NONE',  ( 0.000000000000000000, 0.000000000000000000, 0.1377952755905511584 ) ) ;
#25935=CARTESIAN_POINT ( 'NONE',  ( -0.2230788859036007821, 0.2650812153444458419, 0.1377952755905510474 ) ) ;
#25938=ORIENTED_EDGE ( 'NONE', *, *, #3005, .T. ) ;
#25948=DIRECTION ( 'NONE',  ( 0.000000000000000000, 1.000000000000000000, 0.000000000000000000 ) ) ;
#25964=ORIENTED_EDGE ( 'NONE', *, *, #21081, .F. ) ;
#25989=ORIENTED_EDGE ( 'NONE', *, *, #23764, .T. ) ;
#26003=DIRECTION ( 'NONE',  ( 0.000000000000000000, -1.000000000000000000, 0.000000000000000000 ) ) ;
#26008=CARTESIAN_POINT ( 'NONE',  ( -0.0005189969344232283309, 0.3771649972486724733, 0.1992125984251968684 ) ) ;
#26010=CARTESIAN_POINT ( 'NONE',  ( -0.2420394123212937232, 0.2892587550802429575, 0.07637795275590551769 ) ) ;
#26025=DIRECTION ( 'NONE',  ( 0.000000000000000000, 0.000000000000000000, 1.000000000000000000 ) ) ;
#26035=CARTESIAN_POINT ( 'NONE',  ( -0.0005189969344232283309, 0.3771649972486724733, 0.07637795275590551769 ) ) ;
#26036=CARTESIAN_POINT ( 'NONE',  ( 0.1694923354752467248, -0.4674199084428152240, 0.1140743250954091431 ) ) ;
#26048=AXIS2_PLACEMENT_3D ( 'NONE', #25012, #12156, #18645 ) ;
#26057=DIRECTION ( 'NONE',  ( 0.000000000000000000, 1.000000000000000000, 0.000000000000000000 ) ) ;
#26092=ADVANCED_FACE ( 'NONE', ( #23757, #16577 ), #15559, .T. ) ;
#26098=EDGE_CURVE ( 'NONE', #11701, #21231, #23274, .T. ) ;
#26117=DIRECTION ( 'NONE',  ( -1.000000000000000000, 1.224646799147353454E-16, 0.000000000000000000 ) ) ;
#26121=EDGE_LOOP ( 'NONE', ( #10477, #9682, #15716, #881, #19610, #11140 ) ) ;
#26131=ORIENTED_EDGE ( 'NONE', *, *, #25526, .T. ) ;
#26136=ORIENTED_EDGE ( 'NONE', *, *, #25029, .F. ) ;
#26141=B_SPLINE_CURVE_WITH_KNOTS ( 'NONE', 3,
 ( #27020, #20092, #15850, #19956, #610, #15722 ),
 .UNSPECIFIED., .F., .F.,
 ( 4, 2, 4 ),
 ( 0.5000000000000000000, 0.7500000000000000000, 1.000000000000000000 ),
 .UNSPECIFIED. ) ;
#26142=CARTESIAN_POINT ( 'NONE',  ( 0.4167985568850881561, 0.07349283109919291235, 0.1377952755905511861 ) ) ;
#26144=CARTESIAN_POINT ( 'NONE',  ( 0.4897507849329837404, 0.08575075074624730065, 0.1615162260786077997 ) ) ;
#26162=CARTESIAN_POINT ( 'NONE',  ( 0.3713448905834433322, 0.06600512665679410251, 0.07637795275590551769 ) ) ;
#26169=CARTESIAN_POINT ( 'NONE',  ( 0.3771653543307086909, 0.000000000000000000, 0.1992125984251968684 ) ) ;
#26170=B_SPLINE_CURVE_WITH_KNOTS ( 'NONE', 3,
 ( #26887, #7537, #27182, #24904, #17962, #26600, #22793, #9930, #16019, #15746 ),
 .UNSPECIFIED., .F., .F.,
 ( 4, 2, 2, 2, 4 ),
 ( 0.000000000000000000, 0.2499999999999998335, 0.4999999999999996669, 0.7499999999999997780, 1.000000000000000000 ),
 .UNSPECIFIED. ) ;
#26174=DIRECTION ( 'NONE',  ( 1.224646799147353207E-16, 1.000000000000000000, -0.000000000000000000 ) ) ;
#26176=CARTESIAN_POINT ( 'NONE',  ( -4.618943439303797186E-17, -0.3771653543307086909, 0.2374015748031496065 ) ) ;
#26179=VERTEX_POINT ( 'NONE', #2399 ) ;
#26185=CARTESIAN_POINT ( 'NONE',  ( 0.000000000000000000, 0.000000000000000000, 0.07637795275590551769 ) ) ;
#26213=ORIENTED_EDGE ( 'NONE', *, *, #24508, .F. ) ;
#26216=CARTESIAN_POINT ( 'NONE',  ( 0.000000000000000000, 0.000000000000000000, -3.278217716535432842E-17 ) ) ;
#26221=CARTESIAN_POINT ( 'NONE',  ( 0.2428345617565153547, 0.2885915454824177218, 0.07637795275590551769 ) ) ;
#26223=ORIENTED_EDGE ( 'NONE', *, *, #1134, .T. ) ;
#26231=ORIENTED_EDGE ( 'NONE', *, *, #13343, .T. ) ;
#26235=AXIS2_PLACEMENT_3D ( 'NONE', #14594, #1705, #14877 ) ;
#26245=EDGE_CURVE ( 'NONE', #3330, #14826, #10170, .T. ) ;
#26249=EDGE_CURVE ( 'NONE', #14009, #3213, #3877, .T. ) ;
#26256=SHAPE_REPRESENTATION_RELATIONSHIP ( 'NONE' , 'NONE' ,  #26684, #10670 ) ;
#26265=VERTEX_POINT ( 'NONE', #18331 ) ;
#26270=CYLINDRICAL_SURFACE ( 'NONE', #6683, 0.3771653543307086909 ) ;
#26274=CARTESIAN_POINT ( 'NONE',  ( 0.4716107359500099072, 0.08256389912644751528, 0.08349695147423491504 ) ) ;
#26275=CARTESIAN_POINT ( 'NONE',  ( -0.2421724791772047192, 0.2891474103999575052, 0.07637630750536809898 ) ) ;
#26292=CARTESIAN_POINT ( 'NONE',  ( -0.2230788859036007821, 0.2650812153444458419, 0.1377952755905510474 ) ) ;
#26295=FILL_AREA_STYLE ('',( #2289 ) ) ;
#26302=DIRECTION ( 'NONE',  ( 1.000000000000000000, 0.000000000000000000, 0.000000000000000000 ) ) ;
#26309=ORIENTED_EDGE ( 'NONE', *, *, #27470, .F. ) ;
#26313=CARTESIAN_POINT ( 'NONE',  ( 0.3132247436407415431, 0.3723693495133243436, 0.09284957166292857889 ) ) ;
#26332=CARTESIAN_POINT ( 'NONE',  ( 0.4061284506583976994, -0.2351468520617074898, 0.1992125984251968684 ) ) ;
#26363=VERTEX_POINT ( 'NONE', #11926 ) ;
#26389=EDGE_CURVE ( 'NONE', #6801, #14102, #1614, .T. ) ;
#26410=CARTESIAN_POINT ( 'NONE',  ( 0.0005789221761214173069, 0.4692909815006417462, 0.07637795275590551769 ) ) ;
#26418=B_SPLINE_CURVE_WITH_KNOTS ( 'NONE', 3,
 ( #15564, #959, #24162, #9546, #23902, #20302 ),
 .UNSPECIFIED., .F., .F.,
 ( 4, 2, 4 ),
 ( 0.7157687286427140139, 0.7172350147555670574, 0.7187013008684189908 ),
 .UNSPECIFIED. ) ;
#26420=ADVANCED_FACE ( 'NONE', ( #6403 ), #1179, .F. ) ;
#26424=ORIENTED_EDGE ( 'NONE', *, *, #5259, .T. ) ;
#26472=ORIENTED_EDGE ( 'NONE', *, *, #10864, .F. ) ;
#26484=DIRECTION ( 'NONE',  ( 1.000000000000000000, 0.000000000000000000, 0.000000000000000000 ) ) ;
#26507=CARTESIAN_POINT ( 'NONE',  ( -0.4167985568850881561, 0.07349283109919310664, 0.1377952755905511861 ) ) ;
#26509=CARTESIAN_POINT ( 'NONE',  ( 0.000000000000000000, 0.000000000000000000, 0.1377952755905511861 ) ) ;
#26518=CARTESIAN_POINT ( 'NONE',  ( -0.4066108233583291542, -0.2343118354750748089, 0.07637630773773071424 ) ) ;
#26527=CARTESIAN_POINT ( 'NONE',  ( -0.5393700787401575214, 6.677700066216866815E-17, 0.2755905511811023723 ) ) ;
#26531=CARTESIAN_POINT ( 'NONE',  ( 0.000000000000000000, 0.000000000000000000, 0.03818897637795275884 ) ) ;
#26536=CARTESIAN_POINT ( 'NONE',  ( -0.1220886091251831423, -0.3369140789106654932, 0.09506557084502520460 ) ) ;
#26542=CARTESIAN_POINT ( 'NONE',  ( 0.4066108233583291542, -0.2343118354750751975, 0.07637630773773071424 ) ) ;
#26577=B_SPLINE_CURVE_WITH_KNOTS ( 'NONE', 3,
 ( #27587, #1174, #10612, #8503, #14890, #19517 ),
 .UNSPECIFIED., .F., .F.,
 ( 4, 2, 4 ),
 ( 0.2376120521391529850, 0.2390783382518560096, 0.2405446243645580073 ),
 .UNSPECIFIED. ) ;
#26600=CARTESIAN_POINT ( 'NONE',  ( -0.4333114377122877503, -0.2494818589555614918, 0.1259302777237963078 ) ) ;
#26602=CARTESIAN_POINT ( 'NONE',  ( -0.1606879121749082706, -0.4409237942971039881, 0.1992150590373740204 ) ) ;
#26611=ORIENTED_EDGE ( 'NONE', *, *, #23370, .T. ) ;
#26649=EDGE_CURVE ( 'NONE', #10900, #17397, #25083, .T. ) ;
#26656=VERTEX_POINT ( 'NONE', #7927 ) ;
#26667=B_SPLINE_CURVE_WITH_KNOTS ( 'NONE', 3,
 ( #18900, #12560, #3354, #16799, #27678, #20894 ),
 .UNSPECIFIED., .F., .F.,
 ( 4, 2, 4 ),
 ( 0.6902184472752670441, 0.6915327610580700446, 0.6928470748408730451 ),
 .UNSPECIFIED. ) ;
#26684=SHAPE_REPRESENTATION ( 'Deep Groove Ball Bearing 15x28x7', ( #11588 ), #2565 ) ;
#26695=ORIENTED_EDGE ( 'NONE', *, *, #10357, .T. ) ;
#26701=CARTESIAN_POINT ( 'NONE',  ( 0.000000000000000000, 0.000000000000000000, 0.2755905511811023723 ) ) ;
#26713=B_SPLINE_CURVE_WITH_KNOTS ( 'NONE', 3,
 ( #3643, #1959, #12421, #5644, #1540, #14271 ),
 .UNSPECIFIED., .F., .F.,
 ( 4, 2, 4 ),
 ( 0.000000000000000000, 0.2500000000000000000, 0.5000000000000000000 ),
 .UNSPECIFIED. ) ;
#26720=CARTESIAN_POINT ( 'NONE',  ( 0.1187185187227448868, -0.3276343780141734441, 0.1166443193830783709 ) ) ;
#26726=DIRECTION ( 'NONE',  ( 0.000000000000000000, 1.000000000000000000, 0.000000000000000000 ) ) ;
#26734=EDGE_LOOP ( 'NONE', ( #8839, #7748, #7355, #22786 ) ) ;
#26742=CIRCLE ( 'NONE', #24052, 0.07677362204724411110 ) ;
#26745=CARTESIAN_POINT ( 'NONE',  ( 0.000000000000000000, 0.000000000000000000, 0.1377952755905511861 ) ) ;
#26785=EDGE_CURVE ( 'NONE', #21657, #10388, #4788, .T. ) ;
#26799=DIRECTION ( 'NONE',  ( 0.000000000000000000, 1.000000000000000000, 0.000000000000000000 ) ) ;
#26805=ORIENTED_EDGE ( 'NONE', *, *, #4633, .F. ) ;
#26810=CARTESIAN_POINT ( 'NONE',  ( 0.0005189969344232283309, 0.3771649972486724733, 0.1992125984251968684 ) ) ;
#26825=CARTESIAN_POINT ( 'NONE',  ( 0.2997912780622382090, -0.1736589463928937538, 0.1377952755905513249 ) ) ;
#26829=AXIS2_PLACEMENT_3D ( 'NONE', #22860, #22710, #1517 ) ;
#26836=CARTESIAN_POINT ( 'NONE',  ( -0.3012109481301850633, 0.3598698725862389813, 0.1992125984251968684 ) ) ;
#26860=EDGE_LOOP ( 'NONE', ( #14742, #14836, #8624, #22226, #25130, #12551 ) ) ;
#26869=DIRECTION ( 'NONE',  ( 0.000000000000000000, 1.000000000000000000, 0.000000000000000000 ) ) ;
#26877=DIRECTION ( 'NONE',  ( 0.000000000000000000, 1.000000000000000000, 0.000000000000000000 ) ) ;
#26878=ORIENTED_EDGE ( 'NONE', *, *, #12083, .T. ) ;
#26882=B_SPLINE_CURVE_WITH_KNOTS ( 'NONE', 3,
 ( #23411, #8283, #6176, #12650, #10384, #19003 ),
 .UNSPECIFIED., .F., .F.,
 ( 4, 2, 4 ),
 ( 0.7157687286427130147, 0.7172350147555660582, 0.7187013008684189908 ),
 .UNSPECIFIED. ) ;
#26883=VERTEX_POINT ( 'NONE', #23614 ) ;
#26887=CARTESIAN_POINT ( 'NONE',  ( -0.4067073728345788064, -0.2341441294389334793, 0.1992125984251968684 ) ) ;
#26890=CARTESIAN_POINT ( 'NONE',  ( 0.3714653163189441387, 0.06532421472592657430, 0.07637549214372835182 ) ) ;
#26893=CARTESIAN_POINT ( 'NONE',  ( 0.4622619257814346572, 0.08092139668567618904, 0.07637795275590551769 ) ) ;
#26918=ORIENTED_EDGE ( 'NONE', *, *, #11834, .F. ) ;
#26923=ORIENTED_EDGE ( 'NONE', *, *, #17561, .F. ) ;
#26931=VERTEX_POINT ( 'NONE', #559 ) ;
#26934=ORIENTED_EDGE ( 'NONE', *, *, #26245, .F. ) ;
#26942=CARTESIAN_POINT ( 'NONE',  ( 0.000000000000000000, 0.000000000000000000, 0.1377952755905511861 ) ) ;
#26946=ORIENTED_EDGE ( 'NONE', *, *, #2035, .T. ) ;
#26951=ORIENTED_EDGE ( 'NONE', *, *, #16272, .T. ) ;
#26952=CARTESIAN_POINT ( 'NONE',  ( -5.747161356628524594E-17, -0.4692913385826771866, 0.2755905511811023723 ) ) ;
#26957=VERTEX_POINT ( 'NONE', #24546 ) ;
#26961=EDGE_CURVE ( 'NONE', #19454, #27117, #6334, .T. ) ;
#26972=EDGE_CURVE ( 'NONE', #16738, #935, #27355, .T. ) ;
#26991=ORIENTED_EDGE ( 'NONE', *, *, #25712, .T. ) ;
#26996=CARTESIAN_POINT ( 'NONE',  ( 0.000000000000000000, 0.000000000000000000, 0.07637795275590551769 ) ) ;
#27012=AXIS2_PLACEMENT_3D ( 'NONE', #23681, #17442, #6853 ) ;
#27020=CARTESIAN_POINT ( 'NONE',  ( 0.0004974201395668471654, 0.3464563358313494934, 0.1377952755905513249 ) ) ;
#27027=AXIS2_PLACEMENT_3D ( 'NONE', #16482, #21144, #1787 ) ;
#27040=CARTESIAN_POINT ( 'NONE',  ( 0.4308867145619961203, -0.2480839813579571174, 0.1615162260888333701 ) ) ;
#27041=AXIS2_PLACEMENT_3D ( 'NONE', #8769, #6381, #17526 ) ;
#27052=EDGE_LOOP ( 'NONE', ( #17219, #25964, #2641, #4080 ) ) ;
#27062=CARTESIAN_POINT ( 'NONE',  ( 0.3432721300517227458, 0.06002180498082428789, 0.1589462317926793600 ) ) ;
#27065=AXIS2_PLACEMENT_3D ( 'NONE', #22186, #2810, #24845 ) ;
#27067=ORIENTED_EDGE ( 'NONE', *, *, #2374, .T. ) ;
#27073=CARTESIAN_POINT ( 'NONE',  ( 0.1293227632562456708, -0.3543012242648960752, 0.1992142436757342316 ) ) ;
#27078=ORIENTED_EDGE ( 'NONE', *, *, #21633, .T. ) ;
#27079=CARTESIAN_POINT ( 'NONE',  ( 0.3665264996331779601, -0.2116141732283464416, 0.1377952755905511861 ) ) ;
#27094=DIRECTION ( 'NONE',  ( 1.000000000000000000, 0.000000000000000000, 0.000000000000000000 ) ) ;
#27096=CARTESIAN_POINT ( 'NONE',  ( -0.3265485372158890010, -0.1887320510662011952, 0.07637549214372854611 ) ) ;
#27107=CARTESIAN_POINT ( 'NONE',  ( -0.4061284506583976994, -0.2351468520617070734, 0.1992125984251968684 ) ) ;
#27117=VERTEX_POINT ( 'NONE', #5200 ) ;
#27148=AXIS2_PLACEMENT_3D ( 'NONE', #16307, #1199, #25335 ) ;
#27149=CARTESIAN_POINT ( 'NONE',  ( -0.0005896702191648601262, 0.4865884552430830845, 0.09284957166429641529 ) ) ;
#27155=VERTEX_POINT ( 'NONE', #27534 ) ;
#27156=CARTESIAN_POINT ( 'NONE',  ( -0.1294857240059045234, -0.3542416573274181357, 0.07637795275590551769 ) ) ;
#27157=EDGE_LOOP ( 'NONE', ( #12730, #24103, #13820, #9153, #24702, #1737, #22157, #10979, #14690, #8368, #10303, #8387, #12584, #690 ) ) ;
#27160=CARTESIAN_POINT ( 'NONE',  ( -0.1293227632562458651, -0.3543012242648960752, 0.1992142436757342316 ) ) ;
#27169=B_SPLINE_CURVE_WITH_KNOTS ( 'NONE', 3,
 ( #21985, #24925, #27062, #9523, #13491, #18120 ),
 .UNSPECIFIED., .F., .F.,
 ( 4, 2, 4 ),
 ( 0.5000000000000000000, 0.7500000000000000000, 1.000000000000000000 ),
 .UNSPECIFIED. ) ;
#27182=CARTESIAN_POINT ( 'NONE',  ( -0.4216927985367120990, -0.2427835582309759432, 0.1827409795191895503 ) ) ;
#27192=AXIS2_PLACEMENT_3D ( 'NONE', #26531, #22172, #24287 ) ;
#27209=ORIENTED_EDGE ( 'NONE', *, *, #19159, .F. ) ;
#27232=CARTESIAN_POINT ( 'NONE',  ( -0.3264619303874877754, -0.1888818218344748001, 0.07637630750536809898 ) ) ;
#27239=EDGE_CURVE ( 'NONE', #8846, #2394, #8040, .T. ) ;
#27240=EDGE_LOOP ( 'NONE', ( #15897, #11253 ) ) ;
#27255=CIRCLE ( 'NONE', #15086, 0.5511811023622047445 ) ;
#27279=CARTESIAN_POINT ( 'NONE',  ( -0.3713448905834433322, 0.06600512665679449109, 0.1992125984251968684 ) ) ;
#27284=CARTESIAN_POINT ( 'NONE',  ( 0.3263749705684267921, -0.1890319631540330891, 0.1992125984251968684 ) ) ;
#27296=CARTESIAN_POINT ( 'NONE',  ( -0.1189624676717062762, -0.3253923344978156829, 0.1478915661218652144 ) ) ;
#27313=ORIENTED_EDGE ( 'NONE', *, *, #24079, .F. ) ;
#27316=CARTESIAN_POINT ( 'NONE',  ( 0.2236164729194649314, 0.2672714825446357856, 0.1166443193927515082 ) ) ;
#27320=CARTESIAN_POINT ( 'NONE',  ( -0.3412792617076849111, 0.05967164814832635888, 0.1377952755905512139 ) ) ;
#27325=CARTESIAN_POINT ( 'NONE',  ( 0.4692913385826771866, 0.000000000000000000, 0.1992125984251968684 ) ) ;
#27333=AXIS2_PLACEMENT_3D ( 'NONE', #14930, #27627, #7857 ) ;
#27355=CIRCLE ( 'NONE', #4768, 0.5393700787401575214 ) ;
#27357=EDGE_LOOP ( 'NONE', ( #4520, #3731, #17106, #22724, #14216 ) ) ;
#27384=VERTEX_POINT ( 'NONE', #26332 ) ;
#27387=CARTESIAN_POINT ( 'NONE',  ( -0.0005056364805145227657, 0.3583524373837457255, 0.09506557084337692587 ) ) ;
#27402=PRODUCT ( 'Deep Groove Ball Bearing 15x28x7', 'Deep Groove Ball Bearing 15x28x7', '', ( #8842 ) ) ;
#27415=CARTESIAN_POINT ( 'NONE',  ( 0.1294857240059045234, -0.3542416573274181357, 0.07637795275590551769 ) ) ;
#27418=DIRECTION ( 'NONE',  ( -0.3420201433256691570, 0.9396926207859084279, 0.000000000000000000 ) ) ;
#27429=ORIENTED_EDGE ( 'NONE', *, *, #5259, .F. ) ;
#27437=ADVANCED_FACE ( 'NONE', ( #11217, #1055 ), #14046, .T. ) ;
#27452=CARTESIAN_POINT ( 'NONE',  ( 0.000000000000000000, 0.000000000000000000, 0.07637795275590551769 ) ) ;
#27459=CARTESIAN_POINT ( 'NONE',  ( 0.3019498226894188897, 0.3592501948415138258, 0.07637630773773071424 ) ) ;
#27470=EDGE_CURVE ( 'NONE', #11701, #20882, #19124, .T. ) ;
#27476=VECTOR ( 'NONE', #7800, 39.37007874015748143 ) ;
#27484=VERTEX_POINT ( 'NONE', #9500 ) ;
#27485=DIRECTION ( 'NONE',  ( 0.000000000000000000, 1.000000000000000000, 0.000000000000000000 ) ) ;
#27495=TOROIDAL_SURFACE ( 'NONE', #12132, 0.4232283464566928832, 0.07677165354330708902 ) ;
#27498=CARTESIAN_POINT ( 'NONE',  ( 0.2720459371704843088, 0.3242117229735830830, 0.1377952755905511861 ) ) ;
#27509=AXIS2_PLACEMENT_3D ( 'NONE', #12334, #16869, #23229 ) ;
#27522=CARTESIAN_POINT ( 'NONE',  ( 0.3412792617076849666, 0.05967164814832576214, 0.1276989850568736595 ) ) ;
#27527=DIRECTION ( 'NONE',  ( 0.000000000000000000, 0.000000000000000000, 1.000000000000000000 ) ) ;
#27530=CARTESIAN_POINT ( 'NONE',  ( 0.3771653543307086909, 0.000000000000000000, 0.07637795275590551769 ) ) ;
#27532=ORIENTED_EDGE ( 'NONE', *, *, #24777, .F. ) ;
#27534=CARTESIAN_POINT ( 'NONE',  ( 0.1294857240059045234, -0.3542416573274181357, 0.1992125984251968684 ) ) ;
#27544=CARTESIAN_POINT ( 'NONE',  ( 0.4621283342336243716, 0.08168108835551360358, 0.1992150590373740204 ) ) ;
#27546=EDGE_CURVE ( 'NONE', #19464, #21657, #14080, .T. ) ;
#27547=TOROIDAL_SURFACE ( 'NONE', #15379, 0.4232283464566928832, 0.07677165354330708902 ) ;
#27551=CARTESIAN_POINT ( 'NONE',  ( -6.750021727583836750E-17, -0.5511811023622047445, 0.01181102362204724393 ) ) ;
#27555=CARTESIAN_POINT ( 'NONE',  ( -0.4621283342336283129, 0.08168108835549449387, 0.07637549214372854611 ) ) ;
#27587=CARTESIAN_POINT ( 'NONE',  ( 0.1599629598573824862, -0.4411872753631803090, 0.07637795275590551769 ) ) ;
#27605=EDGE_CURVE ( 'NONE', #2522, #1348, #2106, .T. ) ;
#27608=CARTESIAN_POINT ( 'NONE',  ( 0.1632039128452630883, -0.4501088385450159879, 0.1920935997052418687 ) ) ;
#27610=CARTESIAN_POINT ( 'NONE',  ( -4.618943439303797186E-17, -0.3771653543307086909, 0.03818897637795275884 ) ) ;
#27620=VERTEX_POINT ( 'NONE', #8762 ) ;
#27621=ORIENTED_EDGE ( 'NONE', *, *, #18511, .F. ) ;
#27624=EDGE_LOOP ( 'NONE', ( #25989, #14994, #15903, #8043 ) ) ;
#27627=DIRECTION ( 'NONE',  ( 0.000000000000000000, 0.000000000000000000, 1.000000000000000000 ) ) ;
#27632=TOROIDAL_SURFACE ( 'NONE', #25429, 0.3070866141732283561, 0.01181102362204724393 ) ;
#27640=EDGE_CURVE ( 'NONE', #8867, #20727, #11566, .T. ) ;
#27646=AXIS2_PLACEMENT_3D ( 'NONE', #27651, #8295, #16912 ) ;
#27649=CARTESIAN_POINT ( 'NONE',  ( 0.3169330146499940715, -0.1835719822052965799, 0.1910323753043391970 ) ) ;
#27651=CARTESIAN_POINT ( 'NONE',  ( 0.000000000000000000, 0.000000000000000000, 0.1377952755905511861 ) ) ;
#27653=VECTOR ( 'NONE', #22788, 39.37007874015748143 ) ;
#27678=CARTESIAN_POINT ( 'NONE',  ( -0.2427018018350767803, 0.2887032559529634224, 0.1992142436757342316 ) ) ;
#27715=DIRECTION ( 'NONE',  ( 0.000000000000000000, 0.000000000000000000, 1.000000000000000000 ) ) ;
#27716=AXIS2_PLACEMENT_3D ( 'NONE', #8228, #14461, #16850 ) ;
#27723=EDGE_LOOP ( 'NONE', ( #8235, #23616 ) ) ;
#27730=PLANE ( 'NONE',  #6064 ) ;
#27748=AXIS2_PLACEMENT_3D ( 'NONE', #5609, #14083, #22991 ) ;
#27779=SPHERICAL_SURFACE ( 'NONE', #6968, 0.07677362204724409722 ) ;
#27786=EDGE_CURVE ( 'NONE', #17040, #5138, #14796, .T. ) ;
#27788=CARTESIAN_POINT ( 'NONE',  ( 0.4061284506584276199, -0.2351468520616558922, 0.07637795275590551769 ) ) ;
#27795=SPHERICAL_SURFACE ( 'NONE', #11539, 0.07677362204724409722 ) ;
#27826=EDGE_CURVE ( 'NONE', #18410, #10367, #18403, .T. ) ;
#27844=AXIS2_PLACEMENT_3D ( 'NONE', #20913, #22900, #1414 ) ;
#27848=CARTESIAN_POINT ( 'NONE',  ( 0.3411065095061437402, 0.06065137456822566192, 0.1377952755905510474 ) ) ;
#27854=DIRECTION ( 'NONE',  ( 0.000000000000000000, 0.000000000000000000, 1.000000000000000000 ) ) ;
#27863=EDGE_CURVE ( 'NONE', #9720, #23369, #13852, .T. ) ;
#27875=ORIENTED_EDGE ( 'NONE', *, *, #22850, .T. ) ;
#27882=CARTESIAN_POINT ( 'NONE',  ( 0.0005789221761214173069, 0.4692909815006417462, 0.07637795275590551769 ) ) ;
ENDSEC;
END-ISO-10303-21;
